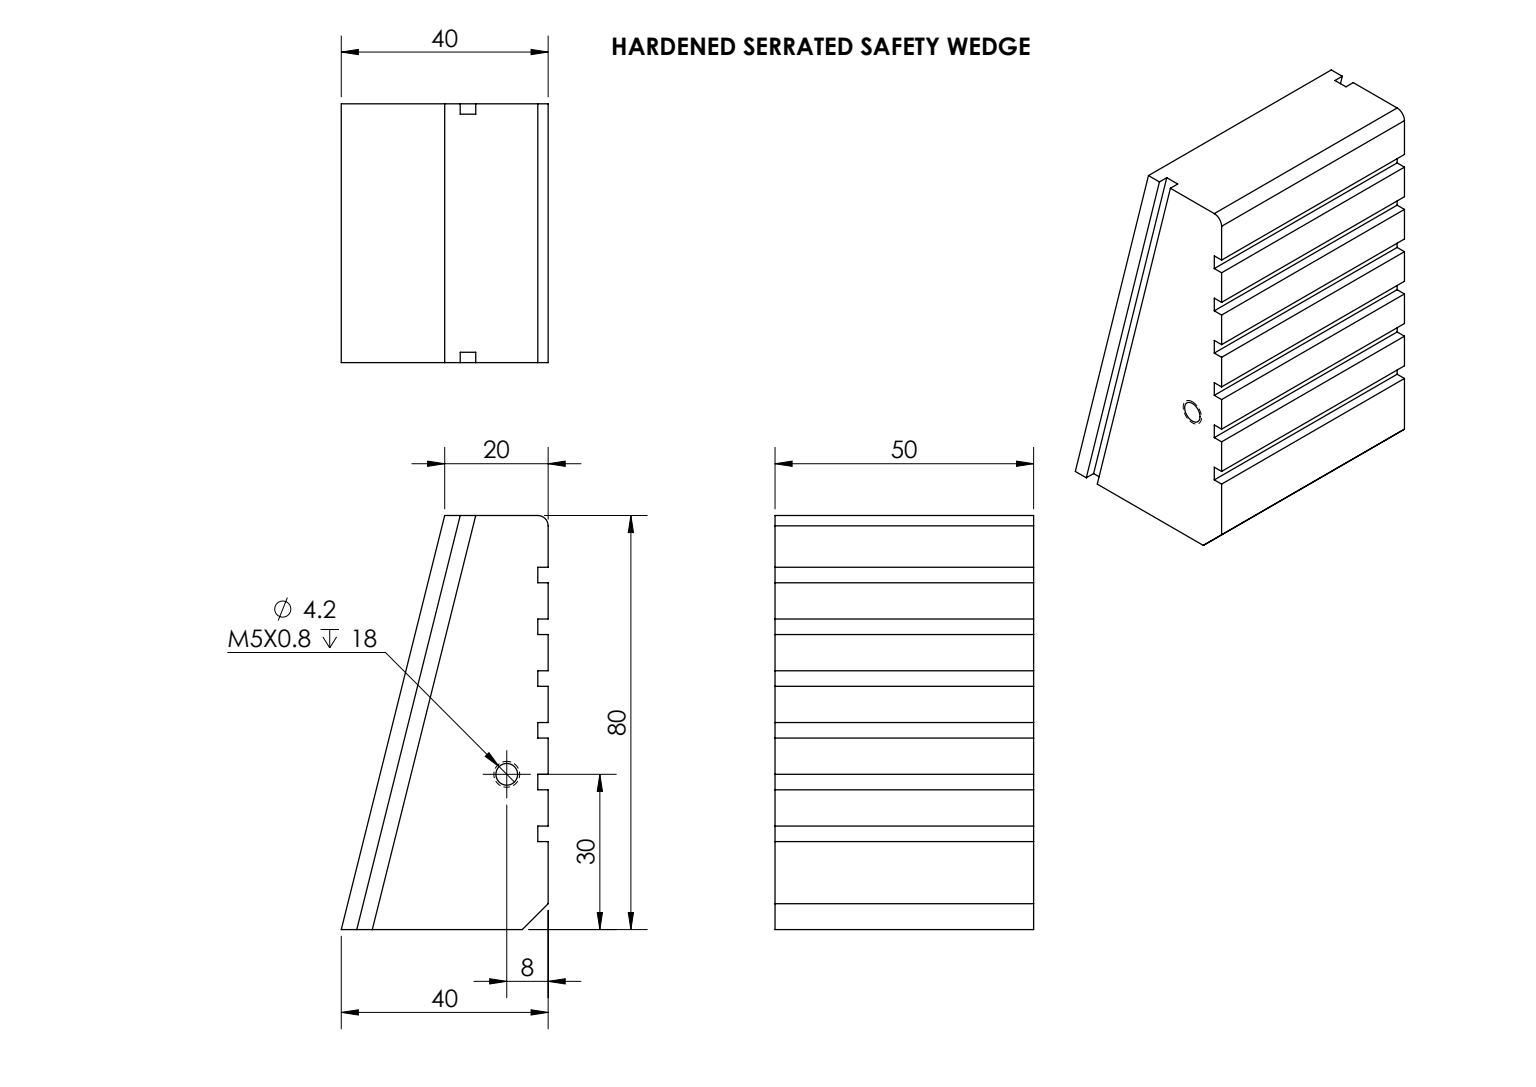
ISO-10303-21;
HEADER;
FILE_DESCRIPTION (('STEP AP214'),
    '1' );
FILE_NAME ('Hardened Serrated Safety Wedge.step',
    '2026-09-24T10:26:00',
    ( '' ),
    ( '' ),
    'SwSTEP 2.0',
    'SolidWorks 2026',
    '' );
FILE_SCHEMA (( 'AUTOMOTIVE_DESIGN' ));
ENDSEC;

DATA;
#10=ORIENTED_EDGE ( 'NONE', *, *, #2223, .T. ) ;
#11=CARTESIAN_POINT ( 'NONE',  ( 36.99999999999999289, 80.00000000000000000, -25.00000000000000000 ) ) ;
#20=DIRECTION ( 'NONE',  ( -1.000000000000000000, 0.000000000000000000, 0.000000000000000000 ) ) ;
#28=FILL_AREA_STYLE ('',( #13572 ) ) ;
#66=LINE ( 'NONE', #136, #7181 ) ;
#72=EDGE_CURVE ( 'NONE', #4842, #5455, #11044, .T. ) ;
#91=DIRECTION ( 'NONE',  ( -0.000000000000000000, -0.000000000000000000, -1.000000000000000000 ) ) ;
#92=ORIENTED_EDGE ( 'NONE', *, *, #1429, .T. ) ;
#97=LINE ( 'NONE', #11278, #533 ) ;
#101=DIRECTION ( 'NONE',  ( 0.000000000000000000, 0.000000000000000000, -1.000000000000000000 ) ) ;
#102=LINE ( 'NONE', #4701, #4263 ) ;
#121=ORIENTED_EDGE ( 'NONE', *, *, #9321, .T. ) ;
#122=DIRECTION ( 'NONE',  ( -0.000000000000000000, -1.000000000000000000, -0.000000000000000000 ) ) ;
#123=ADVANCED_FACE ( 'NONE', ( #3728 ), #1486, .F. ) ;
#124=DIRECTION ( 'NONE',  ( -1.000000000000000000, -1.224646799147353454E-16, 0.000000000000000000 ) ) ;
#126=ORIENTED_EDGE ( 'NONE', *, *, #8617, .F. ) ;
#136=CARTESIAN_POINT ( 'NONE',  ( 19.99999999999999645, 67.00000000000000000, -25.00000000000000000 ) ) ;
#157=AXIS2_PLACEMENT_3D ( 'NONE', #14374, #7610, #12245 ) ;
#161=EDGE_CURVE ( 'NONE', #1060, #1016, #5743, .T. ) ;
#164=ORIENTED_EDGE ( 'NONE', *, *, #6756, .F. ) ;
#166=VECTOR ( 'NONE', #2081, 1000.000000000000000 ) ;
#167=CARTESIAN_POINT ( 'NONE',  ( 0.000000000000000000, 0.000000000000000000, 0.000000000000000000 ) ) ;
#177=DIRECTION ( 'NONE',  ( 0.000000000000000000, 0.000000000000000000, -1.000000000000000000 ) ) ;
#181=VERTEX_POINT ( 'NONE', #10380 ) ;
#197=DIRECTION ( 'NONE',  ( -1.000000000000000000, -0.000000000000000000, -0.000000000000000000 ) ) ;
#209=ORIENTED_EDGE ( 'NONE', *, *, #6776, .T. ) ;
#210=CARTESIAN_POINT ( 'NONE',  ( 22.00000000000000355, 40.00000000000000711, 25.00000000000000000 ) ) ;
#211=ORIENTED_EDGE ( 'NONE', *, *, #12673, .T. ) ;
#223=VECTOR ( 'NONE', #6277, 1000.000000000000000 ) ;
#224=ORIENTED_EDGE ( 'NONE', *, *, #11005, .F. ) ;
#226=ORIENTED_EDGE ( 'NONE', *, *, #6230, .T. ) ;
#228=CARTESIAN_POINT ( 'NONE',  ( 22.00000000000000000, 67.00000000000000000, 25.00000000000000000 ) ) ;
#234=ORIENTED_EDGE ( 'NONE', *, *, #1565, .T. ) ;
#239=EDGE_CURVE ( 'NONE', #9259, #13438, #9577, .T. ) ;
#258=VECTOR ( 'NONE', #7960, 1000.000000000000000 ) ;
#273=FACE_OUTER_BOUND ( 'NONE', #4402, .T. ) ;
#286=ORIENTED_EDGE ( 'NONE', *, *, #14219, .T. ) ;
#294=FACE_OUTER_BOUND ( 'NONE', #7069, .T. ) ;
#297=CARTESIAN_POINT ( 'NONE',  ( 28.00000000000000355, 29.99999999999999645, -6.999999999999992006 ) ) ;
#298=PLANE ( 'NONE',  #9372 ) ;
#301=VECTOR ( 'NONE', #2565, 1000.000000000000000 ) ;
#305=EDGE_CURVE ( 'NONE', #1178, #14168, #3877, .T. ) ;
#311=EDGE_CURVE ( 'NONE', #7235, #651, #5038, .T. ) ;
#329=ORIENTED_EDGE ( 'NONE', *, *, #2055, .F. ) ;
#336=LINE ( 'NONE', #6016, #9990 ) ;
#337=VERTEX_POINT ( 'NONE', #12933 ) ;
#355=CARTESIAN_POINT ( 'NONE',  ( 20.00000000000000000, 70.00000000000000000, 25.00000000000000000 ) ) ;
#373=VERTEX_POINT ( 'NONE', #7643 ) ;
#402=CARTESIAN_POINT ( 'NONE',  ( 20.00000000000000000, 47.00000000000000000, -25.00000000000000000 ) ) ;
#407=DIRECTION ( 'NONE',  ( 0.000000000000000000, 0.000000000000000000, -1.000000000000000000 ) ) ;
#426=VECTOR ( 'NONE', #4169, 1000.000000000000114 ) ;
#429=EDGE_CURVE ( 'NONE', #1264, #5665, #1074, .T. ) ;
#434=VECTOR ( 'NONE', #1179, 1000.000000000000000 ) ;
#435=VERTEX_POINT ( 'NONE', #12201 ) ;
#448=LINE ( 'NONE', #1383, #301 ) ;
#485=CARTESIAN_POINT ( 'NONE',  ( 19.99999999999999645, 57.00000000000000000, 25.00000000000000000 ) ) ;
#509=LINE ( 'NONE', #9432, #9588 ) ;
#511=AXIS2_PLACEMENT_3D ( 'NONE', #2346, #91, #4566 ) ;
#513=LINE ( 'NONE', #8482, #11201 ) ;
#521=CARTESIAN_POINT ( 'NONE',  ( 28.00000000000000355, 29.99999999999999645, -5.738192700042120897 ) ) ;
#533=VECTOR ( 'NONE', #11200, 1000.000000000000000 ) ;
#538=ORIENTED_EDGE ( 'NONE', *, *, #8944, .T. ) ;
#553=FACE_OUTER_BOUND ( 'NONE', #9521, .T. ) ;
#560=LINE ( 'NONE', #11665, #13855 ) ;
#576=PLANE ( 'NONE',  #3995 ) ;
#587=DIRECTION ( 'NONE',  ( -0.2425356250363328581, 0.9701425001453318764, -0.000000000000000000 ) ) ;
#594=LINE ( 'NONE', #11851, #8147 ) ;
#612=ORIENTED_EDGE ( 'NONE', *, *, #11829, .T. ) ;
#618=FACE_OUTER_BOUND ( 'NONE', #7794, .T. ) ;
#634=ORIENTED_EDGE ( 'NONE', *, *, #1889, .T. ) ;
#649=ORIENTED_EDGE ( 'NONE', *, *, #239, .T. ) ;
#651=VERTEX_POINT ( 'NONE', #11316 ) ;
#654=DIRECTION ( 'NONE',  ( 0.7071067811865467956, -0.7071067811865483499, -0.000000000000000000 ) ) ;
#676=VECTOR ( 'NONE', #9454, 1000.000000000000000 ) ;
#678=VECTOR ( 'NONE', #13825, 1000.000000000000000 ) ;
#691=CARTESIAN_POINT ( 'NONE',  ( 30.10000000000000497, 29.99999999999999645, -6.999999999999992006 ) ) ;
#715=CARTESIAN_POINT ( 'NONE',  ( 20.00000000000000000, -5.510910596163090344E-15, 25.00000000000000000 ) ) ;
#718=DIRECTION ( 'NONE',  ( -1.000000000000000000, 0.000000000000000000, 0.000000000000000000 ) ) ;
#719=DIRECTION ( 'NONE',  ( -0.000000000000000000, 1.000000000000000000, 0.000000000000000000 ) ) ;
#721=VERTEX_POINT ( 'NONE', #10426 ) ;
#730=VECTOR ( 'NONE', #6841, 1000.000000000000000 ) ;
#736=ADVANCED_FACE ( 'NONE', ( #5952 ), #4871, .T. ) ;
#741=ORIENTED_EDGE ( 'NONE', *, *, #8946, .F. ) ;
#742=EDGE_CURVE ( 'NONE', #5183, #3543, #1654, .T. ) ;
#744=ORIENTED_EDGE ( 'NONE', *, *, #1270, .T. ) ;
#752=LINE ( 'NONE', #6297, #3942 ) ;
#755=DIRECTION ( 'NONE',  ( 0.9701425001453319874, 0.2425356250363328858, -0.000000000000000000 ) ) ;
#762=DIRECTION ( 'NONE',  ( 0.8571673007021134438, 1.049727191138620051E-16, -0.5150380749100522682 ) ) ;
#777=VERTEX_POINT ( 'NONE', #1804 ) ;
#785=ORIENTED_EDGE ( 'NONE', *, *, #8014, .F. ) ;
#789=FACE_OUTER_BOUND ( 'NONE', #1160, .T. ) ;
#806=PLANE ( 'NONE',  #7277 ) ;
#808=ORIENTED_EDGE ( 'NONE', *, *, #305, .F. ) ;
#809=DIRECTION ( 'NONE',  ( 0.000000000000000000, 0.000000000000000000, -1.000000000000000000 ) ) ;
#815=VERTEX_POINT ( 'NONE', #7418 ) ;
#844=CARTESIAN_POINT ( 'NONE',  ( 20.00000000000000000, 60.00000000000000711, -25.00000000000000000 ) ) ;
#864=CARTESIAN_POINT ( 'NONE',  ( 0.000000000000000000, 0.000000000000000000, 25.00000000000000000 ) ) ;
#869=CARTESIAN_POINT ( 'NONE',  ( 19.99999999999999645, 57.00000000000000000, -25.00000000000000000 ) ) ;
#871=VECTOR ( 'NONE', #14102, 1000.000000000000000 ) ;
#873=LINE ( 'NONE', #3165, #7989 ) ;
#874=CARTESIAN_POINT ( 'NONE',  ( 22.00000000000000355, 30.00000000000000711, 25.00000000000000000 ) ) ;
#882=CARTESIAN_POINT ( 'NONE',  ( 20.00000000000000355, 17.00000000000000000, 25.00000000000000000 ) ) ;
#890=VECTOR ( 'NONE', #3948, 1000.000000000000000 ) ;
#892=FACE_BOUND ( 'NONE', #3702, .T. ) ;
#895=ORIENTED_EDGE ( 'NONE', *, *, #5382, .T. ) ;
#905=EDGE_LOOP ( 'NONE', ( #9782, #10029, #10993, #1163 ) ) ;
#936=EDGE_CURVE ( 'NONE', #1368, #337, #11148, .T. ) ;
#939=ORIENTED_EDGE ( 'NONE', *, *, #7348, .T. ) ;
#941=VECTOR ( 'NONE', #3510, 1000.000000000000000 ) ;
#959=CARTESIAN_POINT ( 'NONE',  ( 56.99999999999997868, -8.673617379884035472E-16, -25.00000000000000000 ) ) ;
#975=PLANE ( 'NONE',  #9030 ) ;
#976=COLOUR_RGB ( '', 0.40784314, 0.44705882, 0.49803922) ;
#1001=ORIENTED_EDGE ( 'NONE', *, *, #8828, .F. ) ;
#1007=EDGE_CURVE ( 'NONE', #8772, #4305, #2374, .T. ) ;
#1014=VECTOR ( 'NONE', #5792, 1000.000000000000000 ) ;
#1016=VERTEX_POINT ( 'NONE', #13577 ) ;
#1024=ORIENTED_EDGE ( 'NONE', *, *, #3965, .T. ) ;
#1030=PLANE ( 'NONE',  #1314 ) ;
#1041=LINE ( 'NONE', #402, #1014 ) ;
#1042=ADVANCED_BREP_SHAPE_REPRESENTATION ( '', ( #6767, #11025 ), #6359 ) ;
#1060=VERTEX_POINT ( 'NONE', #6163 ) ;
#1061=DIRECTION ( 'NONE',  ( 0.000000000000000000, 0.000000000000000000, -1.000000000000000000 ) ) ;
#1073=VERTEX_POINT ( 'NONE', #6075 ) ;
#1074=LINE ( 'NONE', #9718, #12689 ) ;
#1108=LINE ( 'NONE', #3244, #10599 ) ;
#1120=ORIENTED_EDGE ( 'NONE', *, *, #4565, .T. ) ;
#1122=( NAMED_UNIT ( * ) SI_UNIT ( $, .STERADIAN. ) SOLID_ANGLE_UNIT ( ) );
#1127=AXIS2_PLACEMENT_3D ( 'NONE', #10215, #1359, #3582 ) ;
#1153=CARTESIAN_POINT ( 'NONE',  ( 20.00000000000000000, 60.00000000000000711, 25.00000000000000000 ) ) ;
#1160=EDGE_LOOP ( 'NONE', ( #13641, #4625, #1471, #1505 ) ) ;
#1163=ORIENTED_EDGE ( 'NONE', *, *, #13094, .F. ) ;
#1169=CARTESIAN_POINT ( 'NONE',  ( 22.00000000000000000, 70.00000000000000000, 25.00000000000000000 ) ) ;
#1178=VERTEX_POINT ( 'NONE', #7398 ) ;
#1179=DIRECTION ( 'NONE',  ( -1.000000000000000000, -0.000000000000000000, -0.000000000000000000 ) ) ;
#1187=CARTESIAN_POINT ( 'NONE',  ( 20.00000000000000000, -5.510910596163090344E-15, -25.00000000000000000 ) ) ;
#1214=AXIS2_PLACEMENT_3D ( 'NONE', #9472, #13943, #8363 ) ;
#1217=VERTEX_POINT ( 'NONE', #7543 ) ;
#1223=VECTOR ( 'NONE', #11410, 1000.000000000000000 ) ;
#1229=LINE ( 'NONE', #8834, #12194 ) ;
#1241=LINE ( 'NONE', #2558, #4227 ) ;
#1246=EDGE_LOOP ( 'NONE', ( #2231, #9201, #6977, #5095 ) ) ;
#1248=DIRECTION ( 'NONE',  ( -0.000000000000000000, 1.000000000000000000, -0.000000000000000000 ) ) ;
#1264=VERTEX_POINT ( 'NONE', #959 ) ;
#1270=EDGE_CURVE ( 'NONE', #10062, #435, #8650, .T. ) ;
#1290=SURFACE_STYLE_FILL_AREA ( #6856 ) ;
#1311=ORIENTED_EDGE ( 'NONE', *, *, #7811, .F. ) ;
#1313=EDGE_LOOP ( 'NONE', ( #3126, #4583, #612, #8364 ) ) ;
#1314=AXIS2_PLACEMENT_3D ( 'NONE', #9957, #12301, #13335 ) ;
#1322=CARTESIAN_POINT ( 'NONE',  ( 22.00000000000000000, 60.00000000000000711, 25.00000000000000000 ) ) ;
#1323=VECTOR ( 'NONE', #124, 1000.000000000000000 ) ;
#1359=DIRECTION ( 'NONE',  ( -0.000000000000000000, 1.000000000000000000, 0.000000000000000000 ) ) ;
#1361=PLANE ( 'NONE',  #11448 ) ;
#1368=VERTEX_POINT ( 'NONE', #11670 ) ;
#1382=MECHANICAL_DESIGN_GEOMETRIC_PRESENTATION_REPRESENTATION('',(#3971),#9336);
#1383=CARTESIAN_POINT ( 'NONE',  ( 22.00000000000000711, 20.00000000000000355, 25.00000000000000000 ) ) ;
#1388=EDGE_LOOP ( 'NONE', ( #2561, #11617, #939, #10546 ) ) ;
#1429=EDGE_CURVE ( 'NONE', #9259, #815, #12695, .T. ) ;
#1436=CARTESIAN_POINT ( 'NONE',  ( 20.00000000000000000, -5.510910596163090344E-15, -25.00000000000000000 ) ) ;
#1446=ADVANCED_FACE ( 'NONE', ( #10505 ), #13953, .T. ) ;
#1471=ORIENTED_EDGE ( 'NONE', *, *, #8427, .F. ) ;
#1486=CONICAL_SURFACE ( 'NONE', #7542, 2.100000000000000977, 1.029744258676656754 ) ;
#1505=ORIENTED_EDGE ( 'NONE', *, *, #12501, .F. ) ;
#1507=VERTEX_POINT ( 'NONE', #7353 ) ;
#1525=VERTEX_POINT ( 'NONE', #11830 ) ;
#1527=DIRECTION ( 'NONE',  ( -0.2425356250363328581, 0.9701425001453318764, 0.000000000000000000 ) ) ;
#1557=CARTESIAN_POINT ( 'NONE',  ( 20.00000000000000000, 60.00000000000000711, 25.00000000000000000 ) ) ;
#1563=VERTEX_POINT ( 'NONE', #6738 ) ;
#1565=EDGE_CURVE ( 'NONE', #5395, #6157, #7605, .T. ) ;
#1582=DIRECTION ( 'NONE',  ( -1.000000000000000000, 0.000000000000000000, 0.000000000000000000 ) ) ;
#1596=DIRECTION ( 'NONE',  ( -1.000000000000000000, 0.000000000000000000, -0.000000000000000000 ) ) ;
#1598=CARTESIAN_POINT ( 'NONE',  ( 20.00000000000000000, 47.00000000000000000, 25.00000000000000000 ) ) ;
#1600=CARTESIAN_POINT ( 'NONE',  ( 19.99999999999999645, 67.00000000000000000, 25.00000000000000000 ) ) ;
#1634=ORIENTED_EDGE ( 'NONE', *, *, #6804, .T. ) ;
#1639=CARTESIAN_POINT ( 'NONE',  ( 36.99999999999999289, 80.00000000000000000, -25.00000000000000000 ) ) ;
#1644=DIRECTION ( 'NONE',  ( 1.000000000000000000, 0.000000000000000000, 0.000000000000000000 ) ) ;
#1645=VERTEX_POINT ( 'NONE', #8115 ) ;
#1647=EDGE_CURVE ( 'NONE', #9523, #181, #102, .T. ) ;
#1654=LINE ( 'NONE', #12854, #2675 ) ;
#1661=LINE ( 'NONE', #6109, #10008 ) ;
#1673=CARTESIAN_POINT ( 'NONE',  ( 40.00000000000000711, 80.00000000000000000, 25.00000000000000000 ) ) ;
#1675=ORIENTED_EDGE ( 'NONE', *, *, #10881, .F. ) ;
#1680=CARTESIAN_POINT ( 'NONE',  ( 22.00000000000000000, 70.00000000000000000, 25.00000000000000000 ) ) ;
#1685=LINE ( 'NONE', #10684, #5641 ) ;
#1709=PRODUCT ( 'Hardened Serrated Safety Wedge', 'Hardened Serrated Safety Wedge', '', ( #3087 ) ) ;
#1716=CARTESIAN_POINT ( 'NONE',  ( 56.99999999999997868, -8.673617379884035472E-16, 23.00000000000000000 ) ) ;
#1722=VERTEX_POINT ( 'NONE', #12984 ) ;
#1723=CARTESIAN_POINT ( 'NONE',  ( 22.00000000000000000, 70.00000000000000000, 25.00000000000000000 ) ) ;
#1739=CARTESIAN_POINT ( 'NONE',  ( 33.99999999999998579, 80.00000000000000000, 23.00000000000000000 ) ) ;
#1742=CARTESIAN_POINT ( 'NONE',  ( 54.35294117647056567, -1.411764705882362358, 25.00000000000000000 ) ) ;
#1743=EDGE_CURVE ( 'NONE', #4861, #4373, #3896, .T. ) ;
#1745=EDGE_LOOP ( 'NONE', ( #6476, #4758, #12311, #5613 ) ) ;
#1748=DIRECTION ( 'NONE',  ( 0.000000000000000000, 0.000000000000000000, -1.000000000000000000 ) ) ;
#1755=CARTESIAN_POINT ( 'NONE',  ( 22.00000000000000711, 20.00000000000000355, -25.00000000000000000 ) ) ;
#1768=ORIENTED_EDGE ( 'NONE', *, *, #2005, .T. ) ;
#1793=CARTESIAN_POINT ( 'NONE',  ( 57.35294117647057277, -1.411764705882362358, -25.00000000000000000 ) ) ;
#1796=LINE ( 'NONE', #2827, #10774 ) ;
#1804=CARTESIAN_POINT ( 'NONE',  ( 22.00000000000000000, 67.00000000000000000, -25.00000000000000000 ) ) ;
#1809=ADVANCED_FACE ( 'NONE', ( #6293 ), #5056, .F. ) ;
#1815=LINE ( 'NONE', #6338, #5328 ) ;
#1826=LINE ( 'NONE', #1598, #6288 ) ;
#1834=VECTOR ( 'NONE', #2821, 1000.000000000000227 ) ;
#1836=ORIENTED_EDGE ( 'NONE', *, *, #2559, .F. ) ;
#1852=CARTESIAN_POINT ( 'NONE',  ( 57.35294117647057277, -1.411764705882362358, -25.00000000000000000 ) ) ;
#1855=LINE ( 'NONE', #7254, #8774 ) ;
#1878=ORIENTED_EDGE ( 'NONE', *, *, #12626, .F. ) ;
#1883=PLANE ( 'NONE',  #3706 ) ;
#1886=CARTESIAN_POINT ( 'NONE',  ( 57.35294117647057277, -1.411764705882362358, 23.00000000000000000 ) ) ;
#1887=CARTESIAN_POINT ( 'NONE',  ( 20.00000000000000000, 27.00000000000000355, 25.00000000000000000 ) ) ;
#1889=EDGE_CURVE ( 'NONE', #1368, #8027, #8777, .T. ) ;
#1907=ORIENTED_EDGE ( 'NONE', *, *, #5733, .T. ) ;
#1909=ADVANCED_FACE ( 'NONE', ( #5485 ), #13413, .F. ) ;
#1953=AXIS2_PLACEMENT_3D ( 'NONE', #7106, #11430, #5005 ) ;
#1974=CARTESIAN_POINT ( 'NONE',  ( 20.00000000000000000, -5.510910596163090344E-15, -25.00000000000000000 ) ) ;
#1975=CARTESIAN_POINT ( 'NONE',  ( 20.00000000000000000, 78.00000000000000000, -25.00000000000000000 ) ) ;
#1977=FACE_OUTER_BOUND ( 'NONE', #8291, .T. ) ;
#1983=EDGE_CURVE ( 'NONE', #12581, #2621, #1241, .T. ) ;
#2005=EDGE_CURVE ( 'NONE', #9291, #5102, #9129, .T. ) ;
#2008=ORIENTED_EDGE ( 'NONE', *, *, #2079, .T. ) ;
#2009=ORIENTED_EDGE ( 'NONE', *, *, #936, .T. ) ;
#2016=EDGE_CURVE ( 'NONE', #1217, #11907, #9581, .T. ) ;
#2027=VECTOR ( 'NONE', #13139, 1000.000000000000000 ) ;
#2037=PLANE ( 'NONE',  #6947 ) ;
#2055=EDGE_CURVE ( 'NONE', #5455, #14165, #5973, .T. ) ;
#2064=EDGE_CURVE ( 'NONE', #3193, #1507, #9654, .T. ) ;
#2069=LINE ( 'NONE', #1187, #2027 ) ;
#2071=VECTOR ( 'NONE', #122, 1000.000000000000000 ) ;
#2079=EDGE_CURVE ( 'NONE', #3573, #12564, #513, .T. ) ;
#2081=DIRECTION ( 'NONE',  ( -0.000000000000000000, -0.000000000000000000, 1.000000000000000000 ) ) ;
#2084=EDGE_CURVE ( 'NONE', #10580, #1563, #11781, .T. ) ;
#2085=EDGE_CURVE ( 'NONE', #6341, #10817, #1826, .T. ) ;
#2090=EDGE_CURVE ( 'NONE', #9523, #5064, #594, .T. ) ;
#2093=DIRECTION ( 'NONE',  ( 0.000000000000000000, 0.000000000000000000, -1.000000000000000000 ) ) ;
#2098=DIRECTION ( 'NONE',  ( 0.000000000000000000, 0.000000000000000000, -1.000000000000000000 ) ) ;
#2100=VECTOR ( 'NONE', #2190, 1000.000000000000000 ) ;
#2142=CARTESIAN_POINT ( 'NONE',  ( 22.00000000000000000, 70.00000000000000000, -25.00000000000000000 ) ) ;
#2152=DIRECTION ( 'NONE',  ( 0.000000000000000000, 0.000000000000000000, -1.000000000000000000 ) ) ;
#2184=CIRCLE ( 'NONE', #4525, 2.100000000000000977 ) ;
#2190=DIRECTION ( 'NONE',  ( -0.000000000000000000, -1.000000000000000000, -0.000000000000000000 ) ) ;
#2214=VECTOR ( 'NONE', #1061, 1000.000000000000000 ) ;
#2220=CARTESIAN_POINT ( 'NONE',  ( 12.50000000000002132, 12.49999999999999289, -25.00000000000000000 ) ) ;
#2223=EDGE_CURVE ( 'NONE', #4126, #4373, #13031, .T. ) ;
#2231=ORIENTED_EDGE ( 'NONE', *, *, #2064, .F. ) ;
#2232=FACE_OUTER_BOUND ( 'NONE', #11849, .T. ) ;
#2256=CARTESIAN_POINT ( 'NONE',  ( 22.00000000000000000, 70.00000000000000000, 25.00000000000000000 ) ) ;
#2258=EDGE_CURVE ( 'NONE', #5183, #9564, #3081, .T. ) ;
#2275=CARTESIAN_POINT ( 'NONE',  ( 20.00000000000000000, 5.000000000000000000, 25.00000000000000000 ) ) ;
#2287=CARTESIAN_POINT ( 'NONE',  ( 20.00000000000000000, 27.00000000000000355, 25.00000000000000000 ) ) ;
#2314=LINE ( 'NONE', #4532, #1323 ) ;
#2324=LINE ( 'NONE', #6775, #12846 ) ;
#2327=VECTOR ( 'NONE', #2940, 1000.000000000000000 ) ;
#2346=CARTESIAN_POINT ( 'NONE',  ( 28.00000000000000355, 29.99999999999999645, -25.00000000000000000 ) ) ;
#2364=ORIENTED_EDGE ( 'NONE', *, *, #11159, .T. ) ;
#2374=LINE ( 'NONE', #3482, #2214 ) ;
#2377=CARTESIAN_POINT ( 'NONE',  ( 22.00000000000000355, 30.00000000000000711, 25.00000000000000000 ) ) ;
#2378=CARTESIAN_POINT ( 'NONE',  ( 20.00000000000000000, 37.00000000000000711, 25.00000000000000000 ) ) ;
#2379=LINE ( 'NONE', #4720, #7432 ) ;
#2389=ORIENTED_EDGE ( 'NONE', *, *, #9189, .F. ) ;
#2433=DIRECTION ( 'NONE',  ( -0.000000000000000000, 0.000000000000000000, 1.000000000000000000 ) ) ;
#2435=ORIENTED_EDGE ( 'NONE', *, *, #14124, .T. ) ;
#2453=EDGE_LOOP ( 'NONE', ( #7931, #9555, #808, #10717 ) ) ;
#2470=LINE ( 'NONE', #2546, #4243 ) ;
#2476=ORIENTED_EDGE ( 'NONE', *, *, #13211, .F. ) ;
#2480=CARTESIAN_POINT ( 'NONE',  ( 22.00000000000000000, 70.00000000000000000, -25.00000000000000000 ) ) ;
#2489=CARTESIAN_POINT ( 'NONE',  ( 20.00000000000000355, 50.00000000000000000, 25.00000000000000000 ) ) ;
#2492=EDGE_LOOP ( 'NONE', ( #3472, #7425, #6478, #3054 ) ) ;
#2498=ORIENTED_EDGE ( 'NONE', *, *, #7318, .T. ) ;
#2527=DIRECTION ( 'NONE',  ( -0.2425356250363328581, 0.9701425001453318764, 0.000000000000000000 ) ) ;
#2546=CARTESIAN_POINT ( 'NONE',  ( 20.00000000000000355, 30.00000000000000711, 25.00000000000000000 ) ) ;
#2558=CARTESIAN_POINT ( 'NONE',  ( 20.00000000000000000, 60.00000000000000711, -25.00000000000000000 ) ) ;
#2559=EDGE_CURVE ( 'NONE', #6341, #10062, #12622, .T. ) ;
#2561=ORIENTED_EDGE ( 'NONE', *, *, #10392, .F. ) ;
#2565=DIRECTION ( 'NONE',  ( -0.000000000000000000, 1.000000000000000000, -0.000000000000000000 ) ) ;
#2570=ORIENTED_EDGE ( 'NONE', *, *, #2223, .F. ) ;
#2577=ORIENTED_EDGE ( 'NONE', *, *, #8273, .T. ) ;
#2578=DIRECTION ( 'NONE',  ( -1.000000000000000000, 0.000000000000000000, -0.000000000000000000 ) ) ;
#2585=PLANE ( 'NONE',  #1953 ) ;
#2597=CARTESIAN_POINT ( 'NONE',  ( 20.00000000000000355, 40.00000000000000711, -25.00000000000000000 ) ) ;
#2600=VECTOR ( 'NONE', #13843, 1000.000000000000000 ) ;
#2613=DIRECTION ( 'NONE',  ( 0.000000000000000000, -1.000000000000000000, 0.000000000000000000 ) ) ;
#2621=VERTEX_POINT ( 'NONE', #844 ) ;
#2638=DIRECTION ( 'NONE',  ( 1.000000000000000000, 0.000000000000000000, 0.000000000000000000 ) ) ;
#2646=EDGE_CURVE ( 'NONE', #435, #5824, #8675, .T. ) ;
#2663=VECTOR ( 'NONE', #10225, 1000.000000000000000 ) ;
#2675=VECTOR ( 'NONE', #3787, 1000.000000000000000 ) ;
#2680=EDGE_CURVE ( 'NONE', #1178, #5665, #8815, .T. ) ;
#2694=LINE ( 'NONE', #715, #5098 ) ;
#2707=DIRECTION ( 'NONE',  ( -0.000000000000000000, 0.000000000000000000, 1.000000000000000000 ) ) ;
#2731=ORIENTED_EDGE ( 'NONE', *, *, #9196, .T. ) ;
#2735=ORIENTED_EDGE ( 'NONE', *, *, #9535, .T. ) ;
#2754=EDGE_LOOP ( 'NONE', ( #12609, #12486, #4903, #9949, #10444, #785, #12523, #13410, #5775, #4321, #6309, #3499, #649, #13958, #10226, #1836, #226, #164, #12811, #12934, #121, #8467, #8808, #8615, #11419, #2831, #2476, #7743, #10745, #7634 ) ) ;
#2757=AXIS2_PLACEMENT_3D ( 'NONE', #4083, #13073, #6319 ) ;
#2760=VECTOR ( 'NONE', #6987, 1000.000000000000000 ) ;
#2765=PLANE ( 'NONE',  #4916 ) ;
#2770=EDGE_CURVE ( 'NONE', #10977, #12581, #2379, .T. ) ;
#2776=VECTOR ( 'NONE', #10811, 1000.000000000000000 ) ;
#2787=CARTESIAN_POINT ( 'NONE',  ( 22.00000000000000355, 30.00000000000000711, -25.00000000000000000 ) ) ;
#2805=EDGE_CURVE ( 'NONE', #12241, #7901, #10264, .T. ) ;
#2821=DIRECTION ( 'NONE',  ( -0.2425356250363328581, 0.9701425001453318764, -0.000000000000000000 ) ) ;
#2827=CARTESIAN_POINT ( 'NONE',  ( 60.00000000000000000, -6.123233995736768255E-16, -23.00000000000000000 ) ) ;
#2831=ORIENTED_EDGE ( 'NONE', *, *, #4707, .F. ) ;
#2846=CARTESIAN_POINT ( 'NONE',  ( 60.00000000000000000, -6.123233995736768255E-16, -25.00000000000000000 ) ) ;
#2859=CARTESIAN_POINT ( 'NONE',  ( 25.90000000000000213, 29.99999999999999645, -25.00000000000000000 ) ) ;
#2867=DIRECTION ( 'NONE',  ( 0.000000000000000000, 0.000000000000000000, -1.000000000000000000 ) ) ;
#2873=MECHANICAL_DESIGN_GEOMETRIC_PRESENTATION_REPRESENTATION('',(#5426),#12446);
#2904=VECTOR ( 'NONE', #4860, 1000.000000000000000 ) ;
#2907=CARTESIAN_POINT ( 'NONE',  ( 20.00000000000000000, -5.510910596163090344E-15, -25.00000000000000000 ) ) ;
#2922=DIRECTION ( 'NONE',  ( -1.000000000000000000, -0.000000000000000000, -0.000000000000000000 ) ) ;
#2930=FACE_OUTER_BOUND ( 'NONE', #10865, .T. ) ;
#2933=PLANE ( 'NONE',  #9775 ) ;
#2940=DIRECTION ( 'NONE',  ( -0.000000000000000000, -1.000000000000000000, -0.000000000000000000 ) ) ;
#2961=LINE ( 'NONE', #10633, #4986 ) ;
#2978=LINE ( 'NONE', #7347, #9045 ) ;
#2981=DIRECTION ( 'NONE',  ( 1.000000000000000000, 1.224646799147353454E-16, -0.000000000000000000 ) ) ;
#2983=CARTESIAN_POINT ( 'NONE',  ( 20.00000000000000355, 30.00000000000000711, 25.00000000000000000 ) ) ;
#2994=CARTESIAN_POINT ( 'NONE',  ( 20.00000000000000355, 17.00000000000000000, -25.00000000000000000 ) ) ;
#2997=ADVANCED_FACE ( 'NONE', ( #6579 ), #9808, .T. ) ;
#2998=EDGE_CURVE ( 'NONE', #1264, #7901, #10715, .T. ) ;
#3029=FACE_OUTER_BOUND ( 'NONE', #9225, .T. ) ;
#3039=ADVANCED_FACE ( 'NONE', ( #10097 ), #6654, .T. ) ;
#3040=ADVANCED_FACE ( 'NONE', ( #4417 ), #1030, .F. ) ;
#3043=LINE ( 'NONE', #4073, #9736 ) ;
#3054=ORIENTED_EDGE ( 'NONE', *, *, #13277, .F. ) ;
#3062=LINE ( 'NONE', #1739, #6317 ) ;
#3081=LINE ( 'NONE', #13240, #10258 ) ;
#3087=PRODUCT_CONTEXT ( 'NONE', #9795, 'mechanical' ) ;
#3100=LINE ( 'NONE', #13255, #13131 ) ;
#3126=ORIENTED_EDGE ( 'NONE', *, *, #2085, .F. ) ;
#3127=FACE_OUTER_BOUND ( 'NONE', #11935, .T. ) ;
#3131=EDGE_LOOP ( 'NONE', ( #7315, #5168, #9079, #14380, #126, #4095, #11671, #3360, #2498, #9694, #10895, #5389 ) ) ;
#3135=ORIENTED_EDGE ( 'NONE', *, *, #6230, .F. ) ;
#3140=DIRECTION ( 'NONE',  ( 0.000000000000000000, -1.000000000000000000, 0.000000000000000000 ) ) ;
#3162=EDGE_CURVE ( 'NONE', #373, #1264, #3043, .T. ) ;
#3165=CARTESIAN_POINT ( 'NONE',  ( 20.00000000000000000, -5.510910596163090344E-15, -25.00000000000000000 ) ) ;
#3169=DIRECTION ( 'NONE',  ( -1.000000000000000000, 0.000000000000000000, -0.000000000000000000 ) ) ;
#3170=VERTEX_POINT ( 'NONE', #8352 ) ;
#3173=CARTESIAN_POINT ( 'NONE',  ( 22.00000000000000355, 37.00000000000000711, 25.00000000000000000 ) ) ;
#3193=VERTEX_POINT ( 'NONE', #691 ) ;
#3201=DIRECTION ( 'NONE',  ( 0.000000000000000000, -0.000000000000000000, -1.000000000000000000 ) ) ;
#3224=LINE ( 'NONE', #869, #9413 ) ;
#3235=CARTESIAN_POINT ( 'NONE',  ( 22.00000000000000355, 50.00000000000000000, 25.00000000000000000 ) ) ;
#3244=CARTESIAN_POINT ( 'NONE',  ( 22.00000000000000000, 57.00000000000000000, 25.00000000000000000 ) ) ;
#3263=ORIENTED_EDGE ( 'NONE', *, *, #12673, .F. ) ;
#3265=EDGE_LOOP ( 'NONE', ( #10728, #1907, #5085, #7095 ) ) ;
#3278=AXIS2_PLACEMENT_3D ( 'NONE', #8415, #9670, #13047 ) ;
#3280=ADVANCED_FACE ( 'NONE', ( #13207 ), #11072, .T. ) ;
#3288=LINE ( 'NONE', #12492, #11902 ) ;
#3298=EDGE_CURVE ( 'NONE', #4830, #14165, #2069, .T. ) ;
#3308=DIRECTION ( 'NONE',  ( 0.9701425001453319874, 0.2425356250363328858, 0.000000000000000000 ) ) ;
#3323=LINE ( 'NONE', #2220, #5450 ) ;
#3324=ORIENTED_EDGE ( 'NONE', *, *, #4531, .F. ) ;
#3337=DIRECTION ( 'NONE',  ( -0.2425356250363328581, 0.9701425001453318764, 0.000000000000000000 ) ) ;
#3347=CARTESIAN_POINT ( 'NONE',  ( 19.99999999999999645, 57.00000000000000000, 25.00000000000000000 ) ) ;
#3360=ORIENTED_EDGE ( 'NONE', *, *, #4681, .F. ) ;
#3364=ORIENTED_EDGE ( 'NONE', *, *, #9327, .T. ) ;
#3394=ORIENTED_EDGE ( 'NONE', *, *, #10742, .T. ) ;
#3396=CARTESIAN_POINT ( 'NONE',  ( 20.00000000000000000, 80.00000000000000000, 25.00000000000000000 ) ) ;
#3443=ORIENTED_EDGE ( 'NONE', *, *, #13537, .F. ) ;
#3445=ORIENTED_EDGE ( 'NONE', *, *, #5382, .F. ) ;
#3457=PLANE ( 'NONE',  #3704 ) ;
#3472=ORIENTED_EDGE ( 'NONE', *, *, #5559, .F. ) ;
#3477=PLANE ( 'NONE',  #11503 ) ;
#3481=VECTOR ( 'NONE', #11583, 1000.000000000000000 ) ;
#3482=CARTESIAN_POINT ( 'NONE',  ( 20.00000000000000355, 40.00000000000000711, 25.00000000000000000 ) ) ;
#3494=AXIS2_PLACEMENT_3D ( 'NONE', #1742, #9568, #4014 ) ;
#3499=ORIENTED_EDGE ( 'NONE', *, *, #10742, .F. ) ;
#3506=FACE_OUTER_BOUND ( 'NONE', #5037, .T. ) ;
#3510=DIRECTION ( 'NONE',  ( 0.000000000000000000, 0.000000000000000000, -1.000000000000000000 ) ) ;
#3538=AXIS2_PLACEMENT_3D ( 'NONE', #3812, #14322, #11695 ) ;
#3543=VERTEX_POINT ( 'NONE', #14179 ) ;
#3552=DIRECTION ( 'NONE',  ( 1.000000000000000000, 0.000000000000000000, -0.000000000000000000 ) ) ;
#3573=VERTEX_POINT ( 'NONE', #14319 ) ;
#3582=DIRECTION ( 'NONE',  ( 0.000000000000000000, -0.000000000000000000, 1.000000000000000000 ) ) ;
#3588=AXIS2_PLACEMENT_3D ( 'NONE', #8981, #5408, #12220 ) ;
#3619=EDGE_CURVE ( 'NONE', #4830, #337, #12114, .T. ) ;
#3646=LINE ( 'NONE', #4737, #12617 ) ;
#3648=LINE ( 'NONE', #1436, #6034 ) ;
#3661=ORIENTED_EDGE ( 'NONE', *, *, #4029, .T. ) ;
#3698=CARTESIAN_POINT ( 'NONE',  ( 22.00000000000000355, 47.00000000000000000, 25.00000000000000000 ) ) ;
#3702=EDGE_LOOP ( 'NONE', ( #4228, #12719 ) ) ;
#3704=AXIS2_PLACEMENT_3D ( 'NONE', #13832, #7831, #3804 ) ;
#3706=AXIS2_PLACEMENT_3D ( 'NONE', #9926, #3140, #3201 ) ;
#3718=CARTESIAN_POINT ( 'NONE',  ( 20.00000000000000355, 40.00000000000000711, 25.00000000000000000 ) ) ;
#3725=LINE ( 'NONE', #7138, #8206 ) ;
#3728=FACE_OUTER_BOUND ( 'NONE', #8959, .T. ) ;
#3746=ORIENTED_EDGE ( 'NONE', *, *, #429, .T. ) ;
#3767=AXIS2_PLACEMENT_3D ( 'NONE', #3929, #7278, #11755 ) ;
#3773=CARTESIAN_POINT ( 'NONE',  ( 25.90000000000000213, 29.99999999999999645, -6.999999999999992006 ) ) ;
#3783=ORIENTED_EDGE ( 'NONE', *, *, #2005, .F. ) ;
#3787=DIRECTION ( 'NONE',  ( 0.000000000000000000, 0.000000000000000000, -1.000000000000000000 ) ) ;
#3789=ADVANCED_FACE ( 'NONE', ( #10486 ), #2585, .F. ) ;
#3804=DIRECTION ( 'NONE',  ( 0.000000000000000000, -0.000000000000000000, -1.000000000000000000 ) ) ;
#3806=ORIENTED_EDGE ( 'NONE', *, *, #3298, .F. ) ;
#3812=CARTESIAN_POINT ( 'NONE',  ( 60.00000000000000000, -6.123233995736768255E-16, 25.00000000000000000 ) ) ;
#3814=FACE_OUTER_BOUND ( 'NONE', #9176, .T. ) ;
#3837=LINE ( 'NONE', #4997, #676 ) ;
#3877=LINE ( 'NONE', #1673, #5911 ) ;
#3883=DIRECTION ( 'NONE',  ( 0.000000000000000000, 0.000000000000000000, -1.000000000000000000 ) ) ;
#3896=LINE ( 'NONE', #12739, #12186 ) ;
#3913=EDGE_LOOP ( 'NONE', ( #14433, #10649, #12146, #1878 ) ) ;
#3919=VECTOR ( 'NONE', #5955, 1000.000000000000000 ) ;
#3923=EDGE_CURVE ( 'NONE', #12157, #3193, #1855, .T. ) ;
#3924=LINE ( 'NONE', #2597, #2904 ) ;
#3929=CARTESIAN_POINT ( 'NONE',  ( 19.99999999999999645, 67.00000000000000000, 25.00000000000000000 ) ) ;
#3942=VECTOR ( 'NONE', #9599, 1000.000000000000000 ) ;
#3946=CIRCLE ( 'NONE', #10711, 2.100000000000000977 ) ;
#3948=DIRECTION ( 'NONE',  ( 1.000000000000000000, 0.000000000000000000, 0.000000000000000000 ) ) ;
#3965=EDGE_CURVE ( 'NONE', #3170, #9934, #5143, .T. ) ;
#3967=ORIENTED_EDGE ( 'NONE', *, *, #72, .F. ) ;
#3971=STYLED_ITEM ( 'NONE', ( #12209 ), #6767 ) ;
#3995=AXIS2_PLACEMENT_3D ( 'NONE', #5176, #10738, #5250 ) ;
#4007=CARTESIAN_POINT ( 'NONE',  ( 20.00000000000000000, 70.00000000000000000, 25.00000000000000000 ) ) ;
#4014=DIRECTION ( 'NONE',  ( 0.2425356250363328581, -0.9701425001453318764, 0.000000000000000000 ) ) ;
#4029=EDGE_CURVE ( 'NONE', #5022, #8001, #5066, .T. ) ;
#4037=CARTESIAN_POINT ( 'NONE',  ( 22.00000000000000000, 57.00000000000000000, -25.00000000000000000 ) ) ;
#4039=SHAPE_DEFINITION_REPRESENTATION ( #8348, #5343 ) ;
#4043=ORIENTED_EDGE ( 'NONE', *, *, #311, .F. ) ;
#4070=EDGE_CURVE ( 'NONE', #8001, #1525, #11284, .T. ) ;
#4073=CARTESIAN_POINT ( 'NONE',  ( 56.99999999999997868, -9.797174393178845379E-16, 25.00000000000000000 ) ) ;
#4083=CARTESIAN_POINT ( 'NONE',  ( 22.00000000000000355, 30.00000000000000711, 25.00000000000000000 ) ) ;
#4095=ORIENTED_EDGE ( 'NONE', *, *, #5830, .F. ) ;
#4103=CARTESIAN_POINT ( 'NONE',  ( 19.99999999999999645, 67.00000000000000000, 25.00000000000000000 ) ) ;
#4126=VERTEX_POINT ( 'NONE', #7609 ) ;
#4150=CARTESIAN_POINT ( 'NONE',  ( 22.00000000000000711, 17.00000000000000000, 25.00000000000000000 ) ) ;
#4163=CARTESIAN_POINT ( 'NONE',  ( 60.00000000000000000, -6.123233995736768255E-16, 25.00000000000000000 ) ) ;
#4169=DIRECTION ( 'NONE',  ( -0.2425356250363328581, 0.9701425001453318764, 0.000000000000000000 ) ) ;
#4212=DIRECTION ( 'NONE',  ( -0.000000000000000000, 1.000000000000000000, 0.000000000000000000 ) ) ;
#4219=CARTESIAN_POINT ( 'NONE',  ( 54.35294117647056567, -1.411764705882362358, -25.00000000000000000 ) ) ;
#4227=VECTOR ( 'NONE', #11402, 1000.000000000000000 ) ;
#4228=ORIENTED_EDGE ( 'NONE', *, *, #11919, .F. ) ;
#4236=EDGE_CURVE ( 'NONE', #1217, #777, #12455, .T. ) ;
#4243=VECTOR ( 'NONE', #11459, 1000.000000000000000 ) ;
#4244=AXIS2_PLACEMENT_3D ( 'NONE', #7611, #2152, #20 ) ;
#4263=VECTOR ( 'NONE', #4633, 1000.000000000000000 ) ;
#4277=DIRECTION ( 'NONE',  ( -1.000000000000000000, 0.000000000000000000, -0.000000000000000000 ) ) ;
#4284=LINE ( 'NONE', #2142, #8474 ) ;
#4305=VERTEX_POINT ( 'NONE', #10837 ) ;
#4309=APPLICATION_CONTEXT ( 'automotive_design' ) ;
#4321=ORIENTED_EDGE ( 'NONE', *, *, #6443, .F. ) ;
#4351=LINE ( 'NONE', #2489, #1223 ) ;
#4360=VECTOR ( 'NONE', #8651, 1000.000000000000000 ) ;
#4373=VERTEX_POINT ( 'NONE', #7323 ) ;
#4402=EDGE_LOOP ( 'NONE', ( #224, #2364, #6078, #8375 ) ) ;
#4404=ADVANCED_FACE ( 'NONE', ( #3029 ), #13123, .F. ) ;
#4408=ORIENTED_EDGE ( 'NONE', *, *, #2646, .T. ) ;
#4413=DIRECTION ( 'NONE',  ( -0.000000000000000000, -1.000000000000000000, -0.000000000000000000 ) ) ;
#4417=FACE_OUTER_BOUND ( 'NONE', #1745, .T. ) ;
#4448=EDGE_LOOP ( 'NONE', ( #9190, #11549, #7257, #10824 ) ) ;
#4493=ORIENTED_EDGE ( 'NONE', *, *, #8944, .F. ) ;
#4521=DIRECTION ( 'NONE',  ( 0.000000000000000000, -0.000000000000000000, 1.000000000000000000 ) ) ;
#4525=AXIS2_PLACEMENT_3D ( 'NONE', #8204, #7028, #13716 ) ;
#4531=EDGE_CURVE ( 'NONE', #10817, #4305, #873, .T. ) ;
#4532=CARTESIAN_POINT ( 'NONE',  ( 60.00000000000000000, -6.123233995736768255E-16, 23.00000000000000000 ) ) ;
#4543=DIRECTION ( 'NONE',  ( 1.000000000000000000, 0.000000000000000000, 0.000000000000000000 ) ) ;
#4547=EDGE_CURVE ( 'NONE', #6762, #5687, #4557, .T. ) ;
#4557=LINE ( 'NONE', #10019, #10820 ) ;
#4565=EDGE_CURVE ( 'NONE', #7705, #5395, #8918, .T. ) ;
#4566=DIRECTION ( 'NONE',  ( -1.000000000000000000, 0.000000000000000000, 0.000000000000000000 ) ) ;
#4583=ORIENTED_EDGE ( 'NONE', *, *, #2559, .T. ) ;
#4625=ORIENTED_EDGE ( 'NONE', *, *, #8617, .T. ) ;
#4633=DIRECTION ( 'NONE',  ( 0.000000000000000000, 0.000000000000000000, -1.000000000000000000 ) ) ;
#4634=AXIS2_PLACEMENT_3D ( 'NONE', #1322, #2578, #2433 ) ;
#4669=FILL_AREA_STYLE_COLOUR ( '', #10254 ) ;
#4671=DIRECTION ( 'NONE',  ( 0.000000000000000000, 0.000000000000000000, -1.000000000000000000 ) ) ;
#4672=VECTOR ( 'NONE', #10448, 1000.000000000000000 ) ;
#4680=VERTEX_POINT ( 'NONE', #2480 ) ;
#4681=EDGE_CURVE ( 'NONE', #14168, #3573, #7075, .T. ) ;
#4686=CARTESIAN_POINT ( 'NONE',  ( 20.00000000000000000, 80.00000000000000000, 25.00000000000000000 ) ) ;
#4689=FACE_OUTER_BOUND ( 'NONE', #4905, .T. ) ;
#4701=CARTESIAN_POINT ( 'NONE',  ( 19.99999999999999645, 67.00000000000000000, 25.00000000000000000 ) ) ;
#4707=EDGE_CURVE ( 'NONE', #4842, #9976, #6795, .T. ) ;
#4718=LINE ( 'NONE', #11740, #1834 ) ;
#4720=CARTESIAN_POINT ( 'NONE',  ( 22.00000000000000000, 60.00000000000000711, -25.00000000000000000 ) ) ;
#4737=CARTESIAN_POINT ( 'NONE',  ( 33.99999999999998579, 80.00000000000000000, -25.00000000000000000 ) ) ;
#4753=DIRECTION ( 'NONE',  ( -0.000000000000000000, 1.000000000000000000, -0.000000000000000000 ) ) ;
#4755=CARTESIAN_POINT ( 'NONE',  ( 56.99999999999997868, -9.797174393178845379E-16, 25.00000000000000000 ) ) ;
#4758=ORIENTED_EDGE ( 'NONE', *, *, #7735, .T. ) ;
#4762=VECTOR ( 'NONE', #7302, 1000.000000000000000 ) ;
#4767=ORIENTED_EDGE ( 'NONE', *, *, #4707, .T. ) ;
#4785=ADVANCED_FACE ( 'NONE', ( #9508 ), #10872, .F. ) ;
#4818=LINE ( 'NONE', #7074, #12605 ) ;
#4825=CARTESIAN_POINT ( 'NONE',  ( 22.00000000000000355, 47.00000000000000000, 25.00000000000000000 ) ) ;
#4830=VERTEX_POINT ( 'NONE', #11008 ) ;
#4842=VERTEX_POINT ( 'NONE', #5451 ) ;
#4845=ORIENTED_EDGE ( 'NONE', *, *, #14443, .T. ) ;
#4860=DIRECTION ( 'NONE',  ( -1.000000000000000000, -0.000000000000000000, -0.000000000000000000 ) ) ;
#4861=VERTEX_POINT ( 'NONE', #2787 ) ;
#4871=PLANE ( 'NONE',  #5244 ) ;
#4882=CARTESIAN_POINT ( 'NONE',  ( 22.00000000000000355, 30.00000000000000711, 25.00000000000000000 ) ) ;
#4888=ORIENTED_EDGE ( 'NONE', *, *, #14076, .F. ) ;
#4890=LINE ( 'NONE', #11619, #13113 ) ;
#4903=ORIENTED_EDGE ( 'NONE', *, *, #4547, .T. ) ;
#4904=VERTEX_POINT ( 'NONE', #8880 ) ;
#4905=EDGE_LOOP ( 'NONE', ( #8003, #13256, #10, #7280 ) ) ;
#4916=AXIS2_PLACEMENT_3D ( 'NONE', #12490, #13892, #13821 ) ;
#4986=VECTOR ( 'NONE', #12027, 1000.000000000000000 ) ;
#4997=CARTESIAN_POINT ( 'NONE',  ( 20.00000000000000000, 78.00000000000000000, 25.00000000000000000 ) ) ;
#5005=DIRECTION ( 'NONE',  ( 0.2425356250363328581, -0.9701425001453318764, 0.000000000000000000 ) ) ;
#5013=CYLINDRICAL_SURFACE ( 'NONE', #1214, 2.100000000000000977 ) ;
#5022=VERTEX_POINT ( 'NONE', #2378 ) ;
#5037=EDGE_LOOP ( 'NONE', ( #741, #3661, #11875, #1311 ) ) ;
#5038=LINE ( 'NONE', #2859, #4762 ) ;
#5044=DIRECTION ( 'NONE',  ( -0.000000000000000000, -1.000000000000000000, -0.000000000000000000 ) ) ;
#5053=ORIENTED_EDGE ( 'NONE', *, *, #1983, .F. ) ;
#5056=PLANE ( 'NONE',  #3278 ) ;
#5064=VERTEX_POINT ( 'NONE', #1557 ) ;
#5066=LINE ( 'NONE', #6441, #8059 ) ;
#5079=LINE ( 'NONE', #10794, #11376 ) ;
#5085=ORIENTED_EDGE ( 'NONE', *, *, #4565, .F. ) ;
#5095=ORIENTED_EDGE ( 'NONE', *, *, #11919, .T. ) ;
#5097=DIRECTION ( 'NONE',  ( -0.9701425001453319874, -0.2425356250363328858, 0.000000000000000000 ) ) ;
#5098=VECTOR ( 'NONE', #6261, 1000.000000000000000 ) ;
#5101=EDGE_CURVE ( 'NONE', #5665, #12241, #4718, .T. ) ;
#5102=VERTEX_POINT ( 'NONE', #1716 ) ;
#5117=DIRECTION ( 'NONE',  ( 0.000000000000000000, 0.000000000000000000, -1.000000000000000000 ) ) ;
#5127=AXIS2_PLACEMENT_3D ( 'NONE', #12797, #7307, #12645 ) ;
#5143=LINE ( 'NONE', #10850, #4360 ) ;
#5157=FACE_OUTER_BOUND ( 'NONE', #9297, .T. ) ;
#5159=EDGE_LOOP ( 'NONE', ( #7101, #5437, #11398 ) ) ;
#5163=EDGE_LOOP ( 'NONE', ( #3443, #9031, #9692, #6186 ) ) ;
#5168=ORIENTED_EDGE ( 'NONE', *, *, #5510, .T. ) ;
#5176=CARTESIAN_POINT ( 'NONE',  ( 24.99999999999999289, -4.898587196589414604E-15, 25.00000000000000000 ) ) ;
#5183=VERTEX_POINT ( 'NONE', #5222 ) ;
#5193=DIRECTION ( 'NONE',  ( -1.000000000000000000, 0.000000000000000000, 0.000000000000000000 ) ) ;
#5210=DIRECTION ( 'NONE',  ( -1.000000000000000000, -0.000000000000000000, -0.000000000000000000 ) ) ;
#5213=ORIENTED_EDGE ( 'NONE', *, *, #4236, .T. ) ;
#5222=CARTESIAN_POINT ( 'NONE',  ( 24.99999999999999289, -4.898587196589414604E-15, 25.00000000000000000 ) ) ;
#5244=AXIS2_PLACEMENT_3D ( 'NONE', #4007, #8377, #9333 ) ;
#5246=PLANE ( 'NONE',  #3494 ) ;
#5250=DIRECTION ( 'NONE',  ( 0.000000000000000000, 0.000000000000000000, -1.000000000000000000 ) ) ;
#5269=VERTEX_POINT ( 'NONE', #9613 ) ;
#5270=CARTESIAN_POINT ( 'NONE',  ( 22.00000000000000355, 50.00000000000000000, -25.00000000000000000 ) ) ;
#5283=LINE ( 'NONE', #13055, #8719 ) ;
#5285=EDGE_CURVE ( 'NONE', #12157, #7235, #4890, .T. ) ;
#5289=DIRECTION ( 'NONE',  ( -0.000000000000000000, -1.000000000000000000, -0.000000000000000000 ) ) ;
#5299=CARTESIAN_POINT ( 'NONE',  ( 20.00000000000000000, 27.00000000000000355, 25.00000000000000000 ) ) ;
#5315=CARTESIAN_POINT ( 'NONE',  ( 0.000000000000000000, 0.000000000000000000, -25.00000000000000000 ) ) ;
#5328=VECTOR ( 'NONE', #10815, 1000.000000000000000 ) ;
#5337=VECTOR ( 'NONE', #8683, 1000.000000000000000 ) ;
#5343=SHAPE_REPRESENTATION ( 'Hardened Serrated Safety Wedge', ( #11025 ), #6359 ) ;
#5353=DIRECTION ( 'NONE',  ( -0.000000000000000000, 1.000000000000000000, 0.000000000000000000 ) ) ;
#5359=PLANE ( 'NONE',  #10533 ) ;
#5382=EDGE_CURVE ( 'NONE', #373, #6157, #4818, .T. ) ;
#5384=CYLINDRICAL_SURFACE ( 'NONE', #8128, 2.000000000000001776 ) ;
#5389=ORIENTED_EDGE ( 'NONE', *, *, #1565, .F. ) ;
#5393=ADVANCED_FACE ( 'NONE', ( #294 ), #11694, .T. ) ;
#5394=VECTOR ( 'NONE', #11265, 1000.000000000000000 ) ;
#5395=VERTEX_POINT ( 'NONE', #10527 ) ;
#5408=DIRECTION ( 'NONE',  ( 0.000000000000000000, -0.000000000000000000, 1.000000000000000000 ) ) ;
#5413=EDGE_CURVE ( 'NONE', #337, #4861, #509, .T. ) ;
#5416=DIRECTION ( 'NONE',  ( -0.2425356250363328581, 0.9701425001453318764, 0.000000000000000000 ) ) ;
#5426=STYLED_ITEM ( 'NONE', ( #11213 ), #1042 ) ;
#5437=ORIENTED_EDGE ( 'NONE', *, *, #5285, .T. ) ;
#5441=DIRECTION ( 'NONE',  ( 1.000000000000000000, 0.000000000000000000, 0.000000000000000000 ) ) ;
#5443=DIRECTION ( 'NONE',  ( 0.000000000000000000, 0.000000000000000000, -1.000000000000000000 ) ) ;
#5450=VECTOR ( 'NONE', #11131, 1000.000000000000000 ) ;
#5451=CARTESIAN_POINT ( 'NONE',  ( 22.00000000000000711, 20.00000000000000355, 25.00000000000000000 ) ) ;
#5455=VERTEX_POINT ( 'NONE', #1755 ) ;
#5485=FACE_OUTER_BOUND ( 'NONE', #6269, .T. ) ;
#5510=EDGE_CURVE ( 'NONE', #1722, #9071, #10956, .T. ) ;
#5529=ORIENTED_EDGE ( 'NONE', *, *, #8616, .F. ) ;
#5543=DIRECTION ( 'NONE',  ( 1.000000000000000000, 0.000000000000000000, 0.000000000000000000 ) ) ;
#5548=ORIENTED_EDGE ( 'NONE', *, *, #13094, .T. ) ;
#5549=AXIS2_PLACEMENT_3D ( 'NONE', #5315, #1748, #718 ) ;
#5550=CARTESIAN_POINT ( 'NONE',  ( 54.35294117647056567, -1.411764705882362358, -23.00000000000000000 ) ) ;
#5559=EDGE_CURVE ( 'NONE', #11907, #4680, #10150, .T. ) ;
#5571=FACE_OUTER_BOUND ( 'NONE', #12119, .T. ) ;
#5575=DIRECTION ( 'NONE',  ( -0.2425356250363328581, 0.9701425001453318764, 0.000000000000000000 ) ) ;
#5576=( LENGTH_UNIT ( ) NAMED_UNIT ( * ) SI_UNIT ( .MILLI., .METRE. ) );
#5613=ORIENTED_EDGE ( 'NONE', *, *, #13008, .F. ) ;
#5625=EDGE_LOOP ( 'NONE', ( #10950, #3394, #286, #13456 ) ) ;
#5632=CIRCLE ( 'NONE', #7970, 2.100000000000000977 ) ;
#5639=LINE ( 'NONE', #13913, #13321 ) ;
#5641=VECTOR ( 'NONE', #12730, 1000.000000000000000 ) ;
#5662=CARTESIAN_POINT ( 'NONE',  ( 22.00000000000000000, 78.00000000000000000, 25.00000000000000000 ) ) ;
#5665=VERTEX_POINT ( 'NONE', #11027 ) ;
#5687=VERTEX_POINT ( 'NONE', #10283 ) ;
#5696=DIRECTION ( 'NONE',  ( -1.000000000000000000, -0.000000000000000000, -0.000000000000000000 ) ) ;
#5700=CLOSED_SHELL ( 'NONE', ( #123, #9823, #12280, #8861, #13095, #1809, #8687, #6435, #11113, #5725, #11522, #6285, #3040, #4785, #8898, #4404, #1446, #2997, #736, #14155, #5393, #9502, #6232, #7351, #3280, #9273, #9038, #6847, #8187, #3039, #12190, #5990, #7668, #8107, #11634, #7039, #6891, #1909, #11294, #3789, #14110, #13799, #12065, #11354 ) ) ;
#5707=( NAMED_UNIT ( * ) SI_UNIT ( $, .STERADIAN. ) SOLID_ANGLE_UNIT ( ) );
#5709=ORIENTED_EDGE ( 'NONE', *, *, #2064, .T. ) ;
#5723=ORIENTED_EDGE ( 'NONE', *, *, #2770, .T. ) ;
#5725=ADVANCED_FACE ( 'NONE', ( #273 ), #2765, .F. ) ;
#5733=EDGE_CURVE ( 'NONE', #1722, #5395, #3646, .T. ) ;
#5736=CARTESIAN_POINT ( 'NONE',  ( 0.000000000000000000, 0.000000000000000000, 25.00000000000000000 ) ) ;
#5737=LINE ( 'NONE', #12627, #941 ) ;
#5743=LINE ( 'NONE', #210, #2663 ) ;
#5775=ORIENTED_EDGE ( 'NONE', *, *, #2090, .T. ) ;
#5792=DIRECTION ( 'NONE',  ( 1.000000000000000000, 0.000000000000000000, 0.000000000000000000 ) ) ;
#5818=DIRECTION ( 'NONE',  ( -0.8571673007021134438, 0.000000000000000000, -0.5150380749100522682 ) ) ;
#5824=VERTEX_POINT ( 'NONE', #11761 ) ;
#5830=EDGE_CURVE ( 'NONE', #12564, #14306, #3062, .T. ) ;
#5841=EDGE_LOOP ( 'NONE', ( #6121, #1024, #6748, #13725 ) ) ;
#5911=VECTOR ( 'NONE', #587, 1000.000000000000227 ) ;
#5919=DIRECTION ( 'NONE',  ( 0.000000000000000000, 0.000000000000000000, -1.000000000000000000 ) ) ;
#5952=FACE_OUTER_BOUND ( 'NONE', #2492, .T. ) ;
#5955=DIRECTION ( 'NONE',  ( 1.000000000000000000, 0.000000000000000000, 0.000000000000000000 ) ) ;
#5973=LINE ( 'NONE', #10529, #11912 ) ;
#5981=LINE ( 'NONE', #12580, #11274 ) ;
#5990=ADVANCED_FACE ( 'NONE', ( #12262 ), #9991, .T. ) ;
#6016=CARTESIAN_POINT ( 'NONE',  ( 54.35294117647056567, -1.411764705882362358, 25.00000000000000000 ) ) ;
#6033=CARTESIAN_POINT ( 'NONE',  ( 22.00000000000000000, 78.00000000000000000, -25.00000000000000000 ) ) ;
#6034=VECTOR ( 'NONE', #9493, 1000.000000000000000 ) ;
#6037=CARTESIAN_POINT ( 'NONE',  ( 20.00000000000000000, 78.00000000000000000, 25.00000000000000000 ) ) ;
#6045=VECTOR ( 'NONE', #6052, 1000.000000000000000 ) ;
#6046=DIRECTION ( 'NONE',  ( -0.000000000000000000, -1.000000000000000000, -0.000000000000000000 ) ) ;
#6052=DIRECTION ( 'NONE',  ( 1.000000000000000000, 0.000000000000000000, 0.000000000000000000 ) ) ;
#6059=CARTESIAN_POINT ( 'NONE',  ( 20.00000000000000355, 50.00000000000000000, 25.00000000000000000 ) ) ;
#6066=ORIENTED_EDGE ( 'NONE', *, *, #1647, .F. ) ;
#6075=CARTESIAN_POINT ( 'NONE',  ( 22.00000000000000711, 17.00000000000000000, -25.00000000000000000 ) ) ;
#6078=ORIENTED_EDGE ( 'NONE', *, *, #3298, .T. ) ;
#6086=VECTOR ( 'NONE', #12384, 1000.000000000000000 ) ;
#6099=EDGE_CURVE ( 'NONE', #8027, #4861, #10190, .T. ) ;
#6109=CARTESIAN_POINT ( 'NONE',  ( 22.00000000000000355, 40.00000000000000711, 25.00000000000000000 ) ) ;
#6121=ORIENTED_EDGE ( 'NONE', *, *, #14219, .F. ) ;
#6138=DIRECTION ( 'NONE',  ( 0.000000000000000000, -1.000000000000000000, 0.000000000000000000 ) ) ;
#6156=CARTESIAN_POINT ( 'NONE',  ( 20.00000000000000355, 50.00000000000000000, -25.00000000000000000 ) ) ;
#6157=VERTEX_POINT ( 'NONE', #11889 ) ;
#6161=ORIENTED_EDGE ( 'NONE', *, *, #11383, .T. ) ;
#6162=UNCERTAINTY_MEASURE_WITH_UNIT (LENGTH_MEASURE( 1.000000000000000082E-05 ), #5576, 'distance_accuracy_value', 'NONE');
#6163=CARTESIAN_POINT ( 'NONE',  ( 22.00000000000000355, 40.00000000000000711, 25.00000000000000000 ) ) ;
#6180=ORIENTED_EDGE ( 'NONE', *, *, #8242, .T. ) ;
#6186=ORIENTED_EDGE ( 'NONE', *, *, #7735, .F. ) ;
#6207=ORIENTED_EDGE ( 'NONE', *, *, #12626, .T. ) ;
#6213=FACE_OUTER_BOUND ( 'NONE', #5159, .T. ) ;
#6229=CARTESIAN_POINT ( 'NONE',  ( 20.00000000000000711, 20.00000000000000355, -25.00000000000000000 ) ) ;
#6230=EDGE_CURVE ( 'NONE', #6341, #8772, #7546, .T. ) ;
#6232=ADVANCED_FACE ( 'NONE', ( #13141 ), #5359, .T. ) ;
#6253=AXIS2_PLACEMENT_3D ( 'NONE', #8606, #5097, #9498 ) ;
#6256=ORIENTED_EDGE ( 'NONE', *, *, #9790, .T. ) ;
#6261=DIRECTION ( 'NONE',  ( -0.000000000000000000, -1.000000000000000000, -0.000000000000000000 ) ) ;
#6264=LINE ( 'NONE', #9713, #12799 ) ;
#6269=EDGE_LOOP ( 'NONE', ( #209, #2008, #4493, #3783 ) ) ;
#6277=DIRECTION ( 'NONE',  ( 0.000000000000000000, 0.000000000000000000, -1.000000000000000000 ) ) ;
#6285=ADVANCED_FACE ( 'NONE', ( #892, #5571 ), #12167, .T. ) ;
#6288=VECTOR ( 'NONE', #3883, 1000.000000000000000 ) ;
#6293=FACE_OUTER_BOUND ( 'NONE', #6456, .T. ) ;
#6297=CARTESIAN_POINT ( 'NONE',  ( 20.00000000000000000, 37.00000000000000711, -25.00000000000000000 ) ) ;
#6309=ORIENTED_EDGE ( 'NONE', *, *, #3965, .F. ) ;
#6313=EDGE_LOOP ( 'NONE', ( #12345, #744, #4408, #12438 ) ) ;
#6317=VECTOR ( 'NONE', #2922, 1000.000000000000000 ) ;
#6319=DIRECTION ( 'NONE',  ( -0.000000000000000000, 0.000000000000000000, 1.000000000000000000 ) ) ;
#6327=CIRCLE ( 'NONE', #7260, 2.100000000000000977 ) ;
#6328=EDGE_LOOP ( 'NONE', ( #11727, #13455, #12853, #9143 ) ) ;
#6338=CARTESIAN_POINT ( 'NONE',  ( 20.00000000000000000, 37.00000000000000711, 25.00000000000000000 ) ) ;
#6341=VERTEX_POINT ( 'NONE', #11207 ) ;
#6351=FACE_OUTER_BOUND ( 'NONE', #3913, .T. ) ;
#6359=( GEOMETRIC_REPRESENTATION_CONTEXT ( 3 ) GLOBAL_UNCERTAINTY_ASSIGNED_CONTEXT ( ( #6162 ) ) GLOBAL_UNIT_ASSIGNED_CONTEXT ( ( #5576, #9011, #5707 ) ) REPRESENTATION_CONTEXT ( 'NONE', 'WORKASPACE' ) );
#6360=AXIS2_PLACEMENT_3D ( 'NONE', #3396, #8717, #8855 ) ;
#6371=VECTOR ( 'NONE', #10969, 1000.000000000000114 ) ;
#6378=CARTESIAN_POINT ( 'NONE',  ( 20.00000000000000000, -5.510910596163090344E-15, 25.00000000000000000 ) ) ;
#6392=DIRECTION ( 'NONE',  ( 0.000000000000000000, 0.000000000000000000, 1.000000000000000000 ) ) ;
#6402=ORIENTED_EDGE ( 'NONE', *, *, #6099, .F. ) ;
#6416=CARTESIAN_POINT ( 'NONE',  ( 20.00000000000000000, 80.00000000000000000, -25.00000000000000000 ) ) ;
#6434=LINE ( 'NONE', #6156, #10557 ) ;
#6435=ADVANCED_FACE ( 'NONE', ( #3814 ), #7146, .F. ) ;
#6441=CARTESIAN_POINT ( 'NONE',  ( 20.00000000000000000, 37.00000000000000711, 25.00000000000000000 ) ) ;
#6443=EDGE_CURVE ( 'NONE', #9934, #5064, #5639, .T. ) ;
#6446=CARTESIAN_POINT ( 'NONE',  ( 22.00000000000000000, 60.00000000000000711, 25.00000000000000000 ) ) ;
#6456=EDGE_LOOP ( 'NONE', ( #8538, #12170, #13518, #11251 ) ) ;
#6476=ORIENTED_EDGE ( 'NONE', *, *, #2084, .F. ) ;
#6478=ORIENTED_EDGE ( 'NONE', *, *, #13008, .T. ) ;
#6509=EDGE_CURVE ( 'NONE', #9523, #1217, #11286, .T. ) ;
#6511=DIRECTION ( 'NONE',  ( 0.000000000000000000, 0.000000000000000000, -1.000000000000000000 ) ) ;
#6524=DIRECTION ( 'NONE',  ( 0.000000000000000000, 0.000000000000000000, 1.000000000000000000 ) ) ;
#6578=VERTEX_POINT ( 'NONE', #1975 ) ;
#6579=FACE_OUTER_BOUND ( 'NONE', #905, .T. ) ;
#6582=CARTESIAN_POINT ( 'NONE',  ( 22.00000000000000000, 80.00000000000000000, 25.00000000000000000 ) ) ;
#6584=VECTOR ( 'NONE', #1248, 1000.000000000000000 ) ;
#6597=DIRECTION ( 'NONE',  ( 0.000000000000000000, -0.000000000000000000, 1.000000000000000000 ) ) ;
#6606=CARTESIAN_POINT ( 'NONE',  ( 20.00000000000000000, -5.510910596163090344E-15, 25.00000000000000000 ) ) ;
#6621=LINE ( 'NONE', #10063, #2071 ) ;
#6637=DIRECTION ( 'NONE',  ( -1.000000000000000000, 0.000000000000000000, 0.000000000000000000 ) ) ;
#6642=ORIENTED_EDGE ( 'NONE', *, *, #11882, .F. ) ;
#6647=ORIENTED_EDGE ( 'NONE', *, *, #14097, .F. ) ;
#6652=DIRECTION ( 'NONE',  ( 1.000000000000000000, 0.000000000000000000, 0.000000000000000000 ) ) ;
#6654=PLANE ( 'NONE',  #6694 ) ;
#6689=CARTESIAN_POINT ( 'NONE',  ( 20.00000000000000355, 17.00000000000000000, -25.00000000000000000 ) ) ;
#6694=AXIS2_PLACEMENT_3D ( 'NONE', #3235, #4277, #12152 ) ;
#6723=ORIENTED_EDGE ( 'NONE', *, *, #3619, .T. ) ;
#6725=DIRECTION ( 'NONE',  ( 0.000000000000000000, -0.000000000000000000, 1.000000000000000000 ) ) ;
#6728=LINE ( 'NONE', #6582, #10080 ) ;
#6738=CARTESIAN_POINT ( 'NONE',  ( 20.00000000000000000, 70.00000000000000000, 25.00000000000000000 ) ) ;
#6748=ORIENTED_EDGE ( 'NONE', *, *, #10141, .T. ) ;
#6756=EDGE_CURVE ( 'NONE', #1060, #8772, #2324, .T. ) ;
#6762=VERTEX_POINT ( 'NONE', #9039 ) ;
#6767=MANIFOLD_SOLID_BREP ( 'AdvancedHole1', #5700 ) ;
#6768=ORIENTED_EDGE ( 'NONE', *, *, #14124, .F. ) ;
#6775=CARTESIAN_POINT ( 'NONE',  ( 20.00000000000000355, 40.00000000000000711, 25.00000000000000000 ) ) ;
#6776=EDGE_CURVE ( 'NONE', #9291, #3573, #3288, .T. ) ;
#6795=LINE ( 'NONE', #12368, #5394 ) ;
#6804=EDGE_CURVE ( 'NONE', #9644, #13416, #3648, .T. ) ;
#6836=DIRECTION ( 'NONE',  ( -0.000000000000000000, 1.000000000000000000, -0.000000000000000000 ) ) ;
#6841=DIRECTION ( 'NONE',  ( 0.000000000000000000, 0.000000000000000000, -1.000000000000000000 ) ) ;
#6847=ADVANCED_FACE ( 'NONE', ( #9262 ), #13746, .T. ) ;
#6856=FILL_AREA_STYLE ('',( #4669 ) ) ;
#6868=CARTESIAN_POINT ( 'NONE',  ( 22.00000000000000355, 40.00000000000000711, 25.00000000000000000 ) ) ;
#6891=ADVANCED_FACE ( 'NONE', ( #789 ), #5246, .F. ) ;
#6909=ORIENTED_EDGE ( 'NONE', *, *, #2055, .T. ) ;
#6918=FACE_OUTER_BOUND ( 'NONE', #2754, .T. ) ;
#6936=ORIENTED_EDGE ( 'NONE', *, *, #6804, .F. ) ;
#6947=AXIS2_PLACEMENT_3D ( 'NONE', #6868, #13107, #12000 ) ;
#6967=LINE ( 'NONE', #3698, #730 ) ;
#6977=ORIENTED_EDGE ( 'NONE', *, *, #311, .T. ) ;
#6987=DIRECTION ( 'NONE',  ( 0.000000000000000000, 0.000000000000000000, -1.000000000000000000 ) ) ;
#7027=ORIENTED_EDGE ( 'NONE', *, *, #5413, .T. ) ;
#7028=DIRECTION ( 'NONE',  ( -0.000000000000000000, -0.000000000000000000, -1.000000000000000000 ) ) ;
#7039=ADVANCED_FACE ( 'NONE', ( #8679 ), #5384, .T. ) ;
#7046=ORIENTED_EDGE ( 'NONE', *, *, #2680, .F. ) ;
#7061=DIRECTION ( 'NONE',  ( -1.000000000000000000, 0.000000000000000000, 0.000000000000000000 ) ) ;
#7069=EDGE_LOOP ( 'NONE', ( #10727, #12418, #11155, #14032 ) ) ;
#7070=EDGE_CURVE ( 'NONE', #6578, #13498, #6621, .T. ) ;
#7074=CARTESIAN_POINT ( 'NONE',  ( 57.35294117647057277, -1.411764705882362358, -23.00000000000000000 ) ) ;
#7075=LINE ( 'NONE', #4686, #258 ) ;
#7095=ORIENTED_EDGE ( 'NONE', *, *, #14443, .F. ) ;
#7101=ORIENTED_EDGE ( 'NONE', *, *, #3923, .F. ) ;
#7106=CARTESIAN_POINT ( 'NONE',  ( 54.35294117647056567, -1.411764705882362358, -25.00000000000000000 ) ) ;
#7132=( LENGTH_UNIT ( ) NAMED_UNIT ( * ) SI_UNIT ( .MILLI., .METRE. ) );
#7138=CARTESIAN_POINT ( 'NONE',  ( 53.99999999999997868, -1.347111479062091166E-15, 25.00000000000000000 ) ) ;
#7146=PLANE ( 'NONE',  #5127 ) ;
#7149=DIRECTION ( 'NONE',  ( 0.000000000000000000, 0.000000000000000000, -1.000000000000000000 ) ) ;
#7181=VECTOR ( 'NONE', #4543, 1000.000000000000000 ) ;
#7188=CARTESIAN_POINT ( 'NONE',  ( 28.00000000000000355, 29.99999999999999645, -25.00000000000000000 ) ) ;
#7233=CARTESIAN_POINT ( 'NONE',  ( 20.00000000000000000, 5.000000000000000000, -25.00000000000000000 ) ) ;
#7235=VERTEX_POINT ( 'NONE', #3773 ) ;
#7254=CARTESIAN_POINT ( 'NONE',  ( 30.10000000000000497, 29.99999999999999645, -6.999999999999992006 ) ) ;
#7257=ORIENTED_EDGE ( 'NONE', *, *, #2805, .F. ) ;
#7260=AXIS2_PLACEMENT_3D ( 'NONE', #7188, #11895, #12927 ) ;
#7269=ORIENTED_EDGE ( 'NONE', *, *, #5285, .F. ) ;
#7277=AXIS2_PLACEMENT_3D ( 'NONE', #864, #5117, #5193 ) ;
#7278=DIRECTION ( 'NONE',  ( -0.000000000000000000, 1.000000000000000000, 0.000000000000000000 ) ) ;
#7280=ORIENTED_EDGE ( 'NONE', *, *, #11548, .F. ) ;
#7302=DIRECTION ( 'NONE',  ( -0.000000000000000000, -0.000000000000000000, -1.000000000000000000 ) ) ;
#7307=DIRECTION ( 'NONE',  ( 1.000000000000000000, 0.000000000000000000, 0.000000000000000000 ) ) ;
#7315=ORIENTED_EDGE ( 'NONE', *, *, #5733, .F. ) ;
#7316=EDGE_CURVE ( 'NONE', #181, #2621, #8444, .T. ) ;
#7318=EDGE_CURVE ( 'NONE', #14168, #12241, #2978, .T. ) ;
#7323=CARTESIAN_POINT ( 'NONE',  ( 20.00000000000000355, 30.00000000000000711, -25.00000000000000000 ) ) ;
#7347=CARTESIAN_POINT ( 'NONE',  ( 40.00000000000000711, 80.00000000000000000, 25.00000000000000000 ) ) ;
#7348=EDGE_CURVE ( 'NONE', #1645, #1073, #12761, .T. ) ;
#7351=ADVANCED_FACE ( 'NONE', ( #5157 ), #9619, .T. ) ;
#7353=CARTESIAN_POINT ( 'NONE',  ( 30.10000000000000497, 29.99999999999999645, -25.00000000000000000 ) ) ;
#7362=DIRECTION ( 'NONE',  ( 0.000000000000000000, -0.000000000000000000, -1.000000000000000000 ) ) ;
#7366=PLANE ( 'NONE',  #6253 ) ;
#7398=CARTESIAN_POINT ( 'NONE',  ( 60.00000000000000000, -6.123233995736768255E-16, 25.00000000000000000 ) ) ;
#7418=CARTESIAN_POINT ( 'NONE',  ( 19.99999999999999645, 57.00000000000000000, -25.00000000000000000 ) ) ;
#7425=ORIENTED_EDGE ( 'NONE', *, *, #8014, .T. ) ;
#7432=VECTOR ( 'NONE', #6836, 1000.000000000000000 ) ;
#7433=EDGE_CURVE ( 'NONE', #721, #1722, #13215, .T. ) ;
#7541=DIRECTION ( 'NONE',  ( -0.2425356250363328581, 0.9701425001453318764, 0.000000000000000000 ) ) ;
#7542=AXIS2_PLACEMENT_3D ( 'NONE', #11395, #9122, #12365 ) ;
#7543=CARTESIAN_POINT ( 'NONE',  ( 22.00000000000000000, 67.00000000000000000, 25.00000000000000000 ) ) ;
#7546=LINE ( 'NONE', #8653, #11702 ) ;
#7605=LINE ( 'NONE', #10246, #6086 ) ;
#7607=PRODUCT_DEFINITION_CONTEXT ( 'detailed design', #4309, 'design' ) ;
#7609=CARTESIAN_POINT ( 'NONE',  ( 20.00000000000000000, 37.00000000000000711, -25.00000000000000000 ) ) ;
#7610=DIRECTION ( 'NONE',  ( 0.000000000000000000, -1.000000000000000000, 0.000000000000000000 ) ) ;
#7611=CARTESIAN_POINT ( 'NONE',  ( 0.000000000000000000, 0.000000000000000000, -25.00000000000000000 ) ) ;
#7618=LINE ( 'NONE', #9832, #166 ) ;
#7624=AXIS2_PLACEMENT_3D ( 'NONE', #1169, #3169, #14429 ) ;
#7634=ORIENTED_EDGE ( 'NONE', *, *, #8828, .T. ) ;
#7643=CARTESIAN_POINT ( 'NONE',  ( 56.99999999999997868, -1.031959805901694782E-15, -23.00000000000000000 ) ) ;
#7668=ADVANCED_FACE ( 'NONE', ( #7985 ), #12460, .T. ) ;
#7669=ORIENTED_EDGE ( 'NONE', *, *, #14316, .T. ) ;
#7680=CARTESIAN_POINT ( 'NONE',  ( 40.00000000000000711, 80.00000000000000000, 25.00000000000000000 ) ) ;
#7692=VECTOR ( 'NONE', #13194, 1000.000000000000000 ) ;
#7700=ORIENTED_EDGE ( 'NONE', *, *, #5510, .F. ) ;
#7705=VERTEX_POINT ( 'NONE', #12589 ) ;
#7730=SURFACE_STYLE_USAGE ( .BOTH. , #10214 ) ;
#7735=EDGE_CURVE ( 'NONE', #10580, #6578, #3837, .T. ) ;
#7743=ORIENTED_EDGE ( 'NONE', *, *, #14366, .F. ) ;
#7785=DIRECTION ( 'NONE',  ( -0.000000000000000000, 1.000000000000000000, 0.000000000000000000 ) ) ;
#7794=EDGE_LOOP ( 'NONE', ( #895, #6256, #8576, #11738 ) ) ;
#7811=EDGE_CURVE ( 'NONE', #4126, #1525, #752, .T. ) ;
#7831=DIRECTION ( 'NONE',  ( 0.000000000000000000, -1.000000000000000000, 0.000000000000000000 ) ) ;
#7901=VERTEX_POINT ( 'NONE', #11 ) ;
#7922=CARTESIAN_POINT ( 'NONE',  ( 22.00000000000000355, 27.00000000000000355, 25.00000000000000000 ) ) ;
#7931=ORIENTED_EDGE ( 'NONE', *, *, #5101, .T. ) ;
#7943=DIRECTION ( 'NONE',  ( 0.000000000000000000, 0.000000000000000000, -1.000000000000000000 ) ) ;
#7960=DIRECTION ( 'NONE',  ( -1.000000000000000000, -0.000000000000000000, -0.000000000000000000 ) ) ;
#7970=AXIS2_PLACEMENT_3D ( 'NONE', #297, #11554, #12369 ) ;
#7985=FACE_OUTER_BOUND ( 'NONE', #5841, .T. ) ;
#7989=VECTOR ( 'NONE', #4413, 1000.000000000000000 ) ;
#7996=DIRECTION ( 'NONE',  ( -1.000000000000000000, -0.000000000000000000, -0.000000000000000000 ) ) ;
#8001=VERTEX_POINT ( 'NONE', #3173 ) ;
#8003=ORIENTED_EDGE ( 'NONE', *, *, #9321, .F. ) ;
#8005=ORIENTED_EDGE ( 'NONE', *, *, #1007, .F. ) ;
#8014=EDGE_CURVE ( 'NONE', #11907, #1563, #9269, .T. ) ;
#8019=ORIENTED_EDGE ( 'NONE', *, *, #4531, .T. ) ;
#8027=VERTEX_POINT ( 'NONE', #4882 ) ;
#8059=VECTOR ( 'NONE', #10914, 1000.000000000000000 ) ;
#8103=DIRECTION ( 'NONE',  ( 0.000000000000000000, 0.000000000000000000, -1.000000000000000000 ) ) ;
#8107=ADVANCED_FACE ( 'NONE', ( #8997 ), #3457, .T. ) ;
#8115=CARTESIAN_POINT ( 'NONE',  ( 22.00000000000000711, 17.00000000000000000, 25.00000000000000000 ) ) ;
#8128=AXIS2_PLACEMENT_3D ( 'NONE', #5662, #2098, #12980 ) ;
#8138=ORIENTED_EDGE ( 'NONE', *, *, #936, .F. ) ;
#8147=VECTOR ( 'NONE', #5044, 1000.000000000000000 ) ;
#8187=ADVANCED_FACE ( 'NONE', ( #10741 ), #2933, .T. ) ;
#8204=CARTESIAN_POINT ( 'NONE',  ( 28.00000000000000355, 29.99999999999999645, -6.999999999999992006 ) ) ;
#8206=VECTOR ( 'NONE', #12629, 1000.000000000000000 ) ;
#8242=EDGE_CURVE ( 'NONE', #9976, #14165, #10878, .T. ) ;
#8255=LINE ( 'NONE', #12727, #11710 ) ;
#8273=EDGE_CURVE ( 'NONE', #13731, #1368, #9574, .T. ) ;
#8289=DIRECTION ( 'NONE',  ( -0.000000000000000000, -0.000000000000000000, -1.000000000000000000 ) ) ;
#8291=EDGE_LOOP ( 'NONE', ( #538, #13836, #5529, #14320 ) ) ;
#8295=EDGE_LOOP ( 'NONE', ( #3967, #4767, #6180, #329 ) ) ;
#8299=ORIENTED_EDGE ( 'NONE', *, *, #14217, .F. ) ;
#8302=( NAMED_UNIT ( * ) SI_UNIT ( $, .STERADIAN. ) SOLID_ANGLE_UNIT ( ) );
#8336=DIRECTION ( 'NONE',  ( -1.000000000000000000, -0.000000000000000000, -0.000000000000000000 ) ) ;
#8337=EDGE_CURVE ( 'NONE', #5102, #5269, #2314, .T. ) ;
#8348=PRODUCT_DEFINITION_SHAPE ( 'NONE', 'NONE',  #9274 ) ;
#8352=CARTESIAN_POINT ( 'NONE',  ( 22.00000000000000000, 57.00000000000000000, 25.00000000000000000 ) ) ;
#8363=DIRECTION ( 'NONE',  ( -1.000000000000000000, 0.000000000000000000, 0.000000000000000000 ) ) ;
#8364=ORIENTED_EDGE ( 'NONE', *, *, #14279, .F. ) ;
#8375=ORIENTED_EDGE ( 'NONE', *, *, #8242, .F. ) ;
#8377=DIRECTION ( 'NONE',  ( 0.000000000000000000, -1.000000000000000000, 0.000000000000000000 ) ) ;
#8383=DIRECTION ( 'NONE',  ( -0.000000000000000000, 0.000000000000000000, -1.000000000000000000 ) ) ;
#8388=CARTESIAN_POINT ( 'NONE',  ( 20.00000000000000711, 20.00000000000000355, 25.00000000000000000 ) ) ;
#8396=VECTOR ( 'NONE', #14060, 1000.000000000000000 ) ;
#8415=CARTESIAN_POINT ( 'NONE',  ( 20.00000000000000000, -5.510910596163090344E-15, 25.00000000000000000 ) ) ;
#8427=EDGE_CURVE ( 'NONE', #9564, #6762, #336, .T. ) ;
#8443=DIRECTION ( 'NONE',  ( 1.000000000000000000, 1.224646799147353454E-16, 0.000000000000000000 ) ) ;
#8444=LINE ( 'NONE', #2907, #13980 ) ;
#8467=ORIENTED_EDGE ( 'NONE', *, *, #11383, .F. ) ;
#8474=VECTOR ( 'NONE', #8998, 1000.000000000000000 ) ;
#8482=CARTESIAN_POINT ( 'NONE',  ( 36.99999999999999289, 80.00000000000000000, 25.00000000000000000 ) ) ;
#8496=CARTESIAN_POINT ( 'NONE',  ( 20.00000000000000000, -5.510910596163090344E-15, 25.00000000000000000 ) ) ;
#8508=UNCERTAINTY_MEASURE_WITH_UNIT (LENGTH_MEASURE( 1.000000000000000082E-05 ), #7132, 'distance_accuracy_value', 'NONE');
#8512=DIRECTION ( 'NONE',  ( 0.000000000000000000, 0.000000000000000000, -1.000000000000000000 ) ) ;
#8520=ORIENTED_EDGE ( 'NONE', *, *, #6756, .T. ) ;
#8537=LINE ( 'NONE', #2994, #2776 ) ;
#8538=ORIENTED_EDGE ( 'NONE', *, *, #9196, .F. ) ;
#8544=EDGE_CURVE ( 'NONE', #9291, #1178, #5079, .T. ) ;
#8576=ORIENTED_EDGE ( 'NONE', *, *, #2998, .F. ) ;
#8581=VECTOR ( 'NONE', #3337, 1000.000000000000114 ) ;
#8586=CARTESIAN_POINT ( 'NONE',  ( 53.99999999999997868, -1.347111479062091166E-15, 25.00000000000000000 ) ) ;
#8606=CARTESIAN_POINT ( 'NONE',  ( 40.00000000000000711, 80.00000000000000000, 25.00000000000000000 ) ) ;
#8615=ORIENTED_EDGE ( 'NONE', *, *, #8273, .F. ) ;
#8616=EDGE_CURVE ( 'NONE', #5269, #14306, #9622, .T. ) ;
#8617=EDGE_CURVE ( 'NONE', #14306, #6762, #7618, .T. ) ;
#8619=AXIS2_PLACEMENT_3D ( 'NONE', #3718, #2613, #7362 ) ;
#8650=LINE ( 'NONE', #10913, #9361 ) ;
#8651=DIRECTION ( 'NONE',  ( -0.000000000000000000, 1.000000000000000000, -0.000000000000000000 ) ) ;
#8653=CARTESIAN_POINT ( 'NONE',  ( 20.00000000000000000, -5.510910596163090344E-15, 25.00000000000000000 ) ) ;
#8675=LINE ( 'NONE', #12052, #10477 ) ;
#8679=FACE_OUTER_BOUND ( 'NONE', #5163, .T. ) ;
#8683=DIRECTION ( 'NONE',  ( 0.000000000000000000, 0.000000000000000000, -1.000000000000000000 ) ) ;
#8687=ADVANCED_FACE ( 'NONE', ( #3127 ), #975, .F. ) ;
#8696=CARTESIAN_POINT ( 'NONE',  ( 28.00000000000000355, 29.99999999999999645, -6.999999999999992006 ) ) ;
#8709=ORIENTED_EDGE ( 'NONE', *, *, #7070, .F. ) ;
#8717=DIRECTION ( 'NONE',  ( 0.000000000000000000, -1.000000000000000000, 0.000000000000000000 ) ) ;
#8719=VECTOR ( 'NONE', #14224, 1000.000000000000000 ) ;
#8748=FACE_OUTER_BOUND ( 'NONE', #8295, .T. ) ;
#8772=VERTEX_POINT ( 'NONE', #9115 ) ;
#8774=VECTOR ( 'NONE', #762, 1000.000000000000000 ) ;
#8777=LINE ( 'NONE', #874, #7692 ) ;
#8803=SURFACE_SIDE_STYLE ('',( #8945 ) ) ;
#8808=ORIENTED_EDGE ( 'NONE', *, *, #1889, .F. ) ;
#8815=LINE ( 'NONE', #4163, #8835 ) ;
#8826=ORIENTED_EDGE ( 'NONE', *, *, #14279, .T. ) ;
#8828=EDGE_CURVE ( 'NONE', #13043, #5183, #6264, .T. ) ;
#8834=CARTESIAN_POINT ( 'NONE',  ( 20.00000000000000355, 30.00000000000000711, 25.00000000000000000 ) ) ;
#8835=VECTOR ( 'NONE', #13088, 1000.000000000000000 ) ;
#8846=DIRECTION ( 'NONE',  ( -0.2425356250363328581, 0.9701425001453318764, 0.000000000000000000 ) ) ;
#8855=DIRECTION ( 'NONE',  ( 0.000000000000000000, -0.000000000000000000, -1.000000000000000000 ) ) ;
#8861=ADVANCED_FACE ( 'NONE', ( #14120 ), #9776, .T. ) ;
#8869=ORIENTED_EDGE ( 'NONE', *, *, #10881, .T. ) ;
#8880=CARTESIAN_POINT ( 'NONE',  ( 22.00000000000000355, 47.00000000000000000, -25.00000000000000000 ) ) ;
#8898=ADVANCED_FACE ( 'NONE', ( #12781 ), #7366, .F. ) ;
#8918=LINE ( 'NONE', #5550, #6371 ) ;
#8935=AXIS2_PLACEMENT_3D ( 'NONE', #8496, #10766, #11941 ) ;
#8944=EDGE_CURVE ( 'NONE', #5102, #12564, #13022, .T. ) ;
#8945=SURFACE_STYLE_FILL_AREA ( #28 ) ;
#8946=EDGE_CURVE ( 'NONE', #5022, #4126, #1815, .T. ) ;
#8959=EDGE_LOOP ( 'NONE', ( #7269, #13474, #8869 ) ) ;
#8981=CARTESIAN_POINT ( 'NONE',  ( 22.00000000000000000, 78.00000000000000000, 25.00000000000000000 ) ) ;
#8991=CARTESIAN_POINT ( 'NONE',  ( 20.00000000000000000, 47.00000000000000000, -25.00000000000000000 ) ) ;
#8997=FACE_OUTER_BOUND ( 'NONE', #13568, .T. ) ;
#8998=DIRECTION ( 'NONE',  ( -0.000000000000000000, 1.000000000000000000, -0.000000000000000000 ) ) ;
#9009=ORIENTED_EDGE ( 'NONE', *, *, #2646, .F. ) ;
#9011=( NAMED_UNIT ( * ) PLANE_ANGLE_UNIT ( ) SI_UNIT ( $, .RADIAN. ) );
#9030=AXIS2_PLACEMENT_3D ( 'NONE', #6606, #12107, #5443 ) ;
#9031=ORIENTED_EDGE ( 'NONE', *, *, #12048, .F. ) ;
#9038=ADVANCED_FACE ( 'NONE', ( #6351 ), #2037, .T. ) ;
#9039=CARTESIAN_POINT ( 'NONE',  ( 33.99999999999998579, 80.00000000000000000, 25.00000000000000000 ) ) ;
#9040=CARTESIAN_POINT ( 'NONE',  ( 19.99999999999999645, 57.00000000000000000, 25.00000000000000000 ) ) ;
#9045=VECTOR ( 'NONE', #8289, 1000.000000000000000 ) ;
#9067=CIRCLE ( 'NONE', #10230, 2.000000000000001776 ) ;
#9071=VERTEX_POINT ( 'NONE', #13242 ) ;
#9078=( NAMED_UNIT ( * ) PLANE_ANGLE_UNIT ( ) SI_UNIT ( $, .RADIAN. ) );
#9079=ORIENTED_EDGE ( 'NONE', *, *, #12048, .T. ) ;
#9102=ORIENTED_EDGE ( 'NONE', *, *, #10141, .F. ) ;
#9115=CARTESIAN_POINT ( 'NONE',  ( 20.00000000000000355, 40.00000000000000711, 25.00000000000000000 ) ) ;
#9122=DIRECTION ( 'NONE',  ( -0.000000000000000000, -0.000000000000000000, -1.000000000000000000 ) ) ;
#9129=LINE ( 'NONE', #4755, #223 ) ;
#9143=ORIENTED_EDGE ( 'NONE', *, *, #4681, .T. ) ;
#9176=EDGE_LOOP ( 'NONE', ( #3135, #12375, #8019, #8005 ) ) ;
#9189=EDGE_CURVE ( 'NONE', #181, #777, #66, .T. ) ;
#9190=ORIENTED_EDGE ( 'NONE', *, *, #429, .F. ) ;
#9196=EDGE_CURVE ( 'NONE', #5064, #2621, #11173, .T. ) ;
#9201=ORIENTED_EDGE ( 'NONE', *, *, #13931, .F. ) ;
#9211=CARTESIAN_POINT ( 'NONE',  ( 20.00000000000000355, 50.00000000000000000, 25.00000000000000000 ) ) ;
#9225=EDGE_LOOP ( 'NONE', ( #1634, #211, #6647, #9860 ) ) ;
#9259=VERTEX_POINT ( 'NONE', #9040 ) ;
#9262=FACE_OUTER_BOUND ( 'NONE', #12128, .T. ) ;
#9269=LINE ( 'NONE', #355, #434 ) ;
#9273=ADVANCED_FACE ( 'NONE', ( #3506 ), #11321, .T. ) ;
#9274=PRODUCT_DEFINITION ( 'UNKNOWN', '', #12014, #7607 ) ;
#9291=VERTEX_POINT ( 'NONE', #13609 ) ;
#9297=EDGE_LOOP ( 'NONE', ( #8138, #634, #9642, #13328 ) ) ;
#9321=EDGE_CURVE ( 'NONE', #5022, #13659, #2694, .T. ) ;
#9327=EDGE_CURVE ( 'NONE', #6578, #9071, #9067, .T. ) ;
#9333=DIRECTION ( 'NONE',  ( 0.000000000000000000, -0.000000000000000000, -1.000000000000000000 ) ) ;
#9336=( GEOMETRIC_REPRESENTATION_CONTEXT ( 3 ) GLOBAL_UNCERTAINTY_ASSIGNED_CONTEXT ( ( #8508 ) ) GLOBAL_UNIT_ASSIGNED_CONTEXT ( ( #7132, #11680, #8302 ) ) REPRESENTATION_CONTEXT ( 'NONE', 'WORKASPACE' ) );
#9346=EDGE_CURVE ( 'NONE', #1507, #651, #3946, .T. ) ;
#9353=DIRECTION ( 'NONE',  ( 0.000000000000000000, 0.000000000000000000, -1.000000000000000000 ) ) ;
#9357=VECTOR ( 'NONE', #177, 1000.000000000000000 ) ;
#9358=CARTESIAN_POINT ( 'NONE',  ( 20.00000000000000000, -5.510910596163090344E-15, 25.00000000000000000 ) ) ;
#9361=VECTOR ( 'NONE', #9899, 1000.000000000000000 ) ;
#9363=EDGE_CURVE ( 'NONE', #8001, #1060, #1661, .T. ) ;
#9372=AXIS2_PLACEMENT_3D ( 'NONE', #9358, #2638, #7149 ) ;
#9373=EDGE_CURVE ( 'NONE', #3543, #721, #11604, .T. ) ;
#9413=VECTOR ( 'NONE', #5543, 1000.000000000000000 ) ;
#9417=CARTESIAN_POINT ( 'NONE',  ( 28.00000000000000355, 29.99999999999999645, -25.00000000000000000 ) ) ;
#9432=CARTESIAN_POINT ( 'NONE',  ( 22.00000000000000355, 30.00000000000000711, -25.00000000000000000 ) ) ;
#9454=DIRECTION ( 'NONE',  ( 0.000000000000000000, 0.000000000000000000, -1.000000000000000000 ) ) ;
#9472=CARTESIAN_POINT ( 'NONE',  ( 28.00000000000000355, 29.99999999999999645, -25.00000000000000000 ) ) ;
#9493=DIRECTION ( 'NONE',  ( -0.000000000000000000, -1.000000000000000000, -0.000000000000000000 ) ) ;
#9498=DIRECTION ( 'NONE',  ( 0.2425356250363328581, -0.9701425001453318764, 0.000000000000000000 ) ) ;
#9502=ADVANCED_FACE ( 'NONE', ( #8748 ), #1883, .T. ) ;
#9508=FACE_OUTER_BOUND ( 'NONE', #12909, .T. ) ;
#9521=EDGE_LOOP ( 'NONE', ( #1675, #5709, #12715, #4043 ) ) ;
#9523=VERTEX_POINT ( 'NONE', #4103 ) ;
#9534=UNCERTAINTY_MEASURE_WITH_UNIT (LENGTH_MEASURE( 1.000000000000000082E-05 ), #12320, 'distance_accuracy_value', 'NONE');
#9535=EDGE_CURVE ( 'NONE', #9644, #1073, #8537, .T. ) ;
#9555=ORIENTED_EDGE ( 'NONE', *, *, #7318, .F. ) ;
#9564=VERTEX_POINT ( 'NONE', #11366 ) ;
#9568=DIRECTION ( 'NONE',  ( -0.9701425001453319874, -0.2425356250363328858, 0.000000000000000000 ) ) ;
#9574=LINE ( 'NONE', #1887, #890 ) ;
#9577=LINE ( 'NONE', #10602, #12960 ) ;
#9581=LINE ( 'NONE', #1680, #4672 ) ;
#9588=VECTOR ( 'NONE', #4753, 1000.000000000000000 ) ;
#9599=DIRECTION ( 'NONE',  ( 1.000000000000000000, 0.000000000000000000, 0.000000000000000000 ) ) ;
#9613=CARTESIAN_POINT ( 'NONE',  ( 53.99999999999997868, -1.324077043022348342E-15, 23.00000000000000000 ) ) ;
#9619=PLANE ( 'NONE',  #2757 ) ;
#9622=LINE ( 'NONE', #14107, #8581 ) ;
#9641=DIRECTION ( 'NONE',  ( 0.000000000000000000, -0.000000000000000000, 1.000000000000000000 ) ) ;
#9642=ORIENTED_EDGE ( 'NONE', *, *, #6099, .T. ) ;
#9644=VERTEX_POINT ( 'NONE', #6689 ) ;
#9654=LINE ( 'NONE', #10607, #8396 ) ;
#9667=VECTOR ( 'NONE', #9744, 1000.000000000000000 ) ;
#9670=DIRECTION ( 'NONE',  ( 1.000000000000000000, 0.000000000000000000, 0.000000000000000000 ) ) ;
#9692=ORIENTED_EDGE ( 'NONE', *, *, #9327, .F. ) ;
#9694=ORIENTED_EDGE ( 'NONE', *, *, #2805, .T. ) ;
#9713=CARTESIAN_POINT ( 'NONE',  ( 24.99999999999999289, -4.898587196589414604E-15, 25.00000000000000000 ) ) ;
#9718=CARTESIAN_POINT ( 'NONE',  ( 60.00000000000000000, -6.123233995736768255E-16, -25.00000000000000000 ) ) ;
#9733=DIRECTION ( 'NONE',  ( -0.000000000000000000, 1.000000000000000000, -0.000000000000000000 ) ) ;
#9736=VECTOR ( 'NONE', #8512, 1000.000000000000000 ) ;
#9743=VECTOR ( 'NONE', #5416, 1000.000000000000114 ) ;
#9744=DIRECTION ( 'NONE',  ( -0.000000000000000000, 1.000000000000000000, -0.000000000000000000 ) ) ;
#9775=AXIS2_PLACEMENT_3D ( 'NONE', #12056, #719, #9641 ) ;
#9776=PLANE ( 'NONE',  #5549 ) ;
#9780=VECTOR ( 'NONE', #7996, 1000.000000000000000 ) ;
#9782=ORIENTED_EDGE ( 'NONE', *, *, #4236, .F. ) ;
#9790=EDGE_CURVE ( 'NONE', #6157, #7901, #10491, .T. ) ;
#9795=APPLICATION_CONTEXT ( 'automotive_design' ) ;
#9808=PLANE ( 'NONE',  #7624 ) ;
#9811=ORIENTED_EDGE ( 'NONE', *, *, #1743, .F. ) ;
#9823=ADVANCED_FACE ( 'NONE', ( #553 ), #5013, .F. ) ;
#9832=CARTESIAN_POINT ( 'NONE',  ( 33.99999999999998579, 80.00000000000000000, 25.00000000000000000 ) ) ;
#9860=ORIENTED_EDGE ( 'NONE', *, *, #10392, .T. ) ;
#9892=CARTESIAN_POINT ( 'NONE',  ( 20.00000000000000000, 5.000000000000000000, 25.00000000000000000 ) ) ;
#9895=AXIS2_PLACEMENT_3D ( 'NONE', #1852, #755, #7541 ) ;
#9899=DIRECTION ( 'NONE',  ( -0.000000000000000000, 1.000000000000000000, -0.000000000000000000 ) ) ;
#9917=ORIENTED_EDGE ( 'NONE', *, *, #14217, .T. ) ;
#9920=DIRECTION ( 'NONE',  ( 1.000000000000000000, 0.000000000000000000, 0.000000000000000000 ) ) ;
#9926=CARTESIAN_POINT ( 'NONE',  ( 20.00000000000000711, 20.00000000000000355, 25.00000000000000000 ) ) ;
#9934=VERTEX_POINT ( 'NONE', #6446 ) ;
#9949=ORIENTED_EDGE ( 'NONE', *, *, #13537, .T. ) ;
#9950=VECTOR ( 'NONE', #101, 1000.000000000000000 ) ;
#9954=CARTESIAN_POINT ( 'NONE',  ( 57.35294117647057277, -1.411764705882362358, 25.00000000000000000 ) ) ;
#9957=CARTESIAN_POINT ( 'NONE',  ( 20.00000000000000000, -5.510910596163090344E-15, 25.00000000000000000 ) ) ;
#9964=FACE_OUTER_BOUND ( 'NONE', #3131, .T. ) ;
#9976=VERTEX_POINT ( 'NONE', #10990 ) ;
#9988=CARTESIAN_POINT ( 'NONE',  ( 20.00000000000000000, 27.00000000000000355, -25.00000000000000000 ) ) ;
#9990=VECTOR ( 'NONE', #2527, 1000.000000000000114 ) ;
#9991=PLANE ( 'NONE',  #12868 ) ;
#10002=ORIENTED_EDGE ( 'NONE', *, *, #742, .T. ) ;
#10008=VECTOR ( 'NONE', #10433, 1000.000000000000000 ) ;
#10009=DIRECTION ( 'NONE',  ( -0.000000000000000000, -0.000000000000000000, -1.000000000000000000 ) ) ;
#10019=CARTESIAN_POINT ( 'NONE',  ( 20.00000000000000000, 80.00000000000000000, 25.00000000000000000 ) ) ;
#10029=ORIENTED_EDGE ( 'NONE', *, *, #2016, .T. ) ;
#10031=PLANE ( 'NONE',  #6360 ) ;
#10050=DIRECTION ( 'NONE',  ( 0.000000000000000000, -0.000000000000000000, 1.000000000000000000 ) ) ;
#10062=VERTEX_POINT ( 'NONE', #4825 ) ;
#10063=CARTESIAN_POINT ( 'NONE',  ( 20.00000000000000000, -5.510910596163090344E-15, -25.00000000000000000 ) ) ;
#10080=VECTOR ( 'NONE', #11057, 1000.000000000000000 ) ;
#10097=FACE_OUTER_BOUND ( 'NONE', #6313, .T. ) ;
#10100=FACE_OUTER_BOUND ( 'NONE', #1246, .T. ) ;
#10120=SHAPE_REPRESENTATION_RELATIONSHIP ( 'NONE' , 'NONE' ,  #5343, #1042 ) ;
#10141=EDGE_CURVE ( 'NONE', #9934, #12581, #1685, .T. ) ;
#10150=LINE ( 'NONE', #2256, #10973 ) ;
#10180=ORIENTED_EDGE ( 'NONE', *, *, #14076, .T. ) ;
#10190=LINE ( 'NONE', #2377, #9357 ) ;
#10214=SURFACE_SIDE_STYLE ('',( #1290 ) ) ;
#10215=CARTESIAN_POINT ( 'NONE',  ( 20.00000000000000000, 37.00000000000000711, 25.00000000000000000 ) ) ;
#10225=DIRECTION ( 'NONE',  ( 0.000000000000000000, 0.000000000000000000, -1.000000000000000000 ) ) ;
#10226=ORIENTED_EDGE ( 'NONE', *, *, #1270, .F. ) ;
#10230=AXIS2_PLACEMENT_3D ( 'NONE', #6033, #8383, #7061 ) ;
#10246=CARTESIAN_POINT ( 'NONE',  ( 33.99999999999998579, 80.00000000000000000, -23.00000000000000000 ) ) ;
#10254=COLOUR_RGB ( '', 0.40784314, 0.44705882, 0.49803922) ;
#10258=VECTOR ( 'NONE', #14197, 1000.000000000000000 ) ;
#10264=LINE ( 'NONE', #14461, #9780 ) ;
#10269=ORIENTED_EDGE ( 'NONE', *, *, #11159, .F. ) ;
#10283=CARTESIAN_POINT ( 'NONE',  ( 22.00000000000000000, 80.00000000000000000, 25.00000000000000000 ) ) ;
#10286=DIRECTION ( 'NONE',  ( -0.2425356250363328581, 0.9701425001453318764, 0.000000000000000000 ) ) ;
#10315=PLANE ( 'NONE',  #10785 ) ;
#10321=ORIENTED_EDGE ( 'NONE', *, *, #13458, .T. ) ;
#10322=ORIENTED_EDGE ( 'NONE', *, *, #1007, .T. ) ;
#10335=CARTESIAN_POINT ( 'NONE',  ( 20.00000000000000355, 17.00000000000000000, 25.00000000000000000 ) ) ;
#10380=CARTESIAN_POINT ( 'NONE',  ( 19.99999999999999645, 67.00000000000000000, -25.00000000000000000 ) ) ;
#10392=EDGE_CURVE ( 'NONE', #12770, #9644, #5737, .T. ) ;
#10397=ORIENTED_EDGE ( 'NONE', *, *, #3162, .T. ) ;
#10406=CARTESIAN_POINT ( 'NONE',  ( 20.00000000000000355, 50.00000000000000000, -25.00000000000000000 ) ) ;
#10419=CARTESIAN_POINT ( 'NONE',  ( 33.99999999999998579, 80.00000000000000000, 23.00000000000000000 ) ) ;
#10424=ORIENTED_EDGE ( 'NONE', *, *, #1743, .T. ) ;
#10426=CARTESIAN_POINT ( 'NONE',  ( 53.99999999999997868, -1.324077043022348342E-15, -25.00000000000000000 ) ) ;
#10433=DIRECTION ( 'NONE',  ( -0.000000000000000000, 1.000000000000000000, -0.000000000000000000 ) ) ;
#10444=ORIENTED_EDGE ( 'NONE', *, *, #2084, .T. ) ;
#10445=CARTESIAN_POINT ( 'NONE',  ( 22.00000000000000711, 20.00000000000000355, 25.00000000000000000 ) ) ;
#10448=DIRECTION ( 'NONE',  ( -0.000000000000000000, 1.000000000000000000, -0.000000000000000000 ) ) ;
#10477=VECTOR ( 'NONE', #2093, 1000.000000000000000 ) ;
#10486=FACE_OUTER_BOUND ( 'NONE', #3265, .T. ) ;
#10491=LINE ( 'NONE', #1639, #3481 ) ;
#10505=FACE_OUTER_BOUND ( 'NONE', #14463, .T. ) ;
#10511=VECTOR ( 'NONE', #11923, 1000.000000000000000 ) ;
#10527=CARTESIAN_POINT ( 'NONE',  ( 33.99999999999998579, 80.00000000000000000, -23.00000000000000000 ) ) ;
#10529=CARTESIAN_POINT ( 'NONE',  ( 20.00000000000000711, 20.00000000000000355, -25.00000000000000000 ) ) ;
#10531=CARTESIAN_POINT ( 'NONE',  ( 20.00000000000000000, -5.510910596163090344E-15, 25.00000000000000000 ) ) ;
#10533=AXIS2_PLACEMENT_3D ( 'NONE', #2287, #4212, #6597 ) ;
#10546=ORIENTED_EDGE ( 'NONE', *, *, #9535, .F. ) ;
#10549=AXIS2_PLACEMENT_3D ( 'NONE', #14201, #2867, #13036 ) ;
#10550=ORIENTED_EDGE ( 'NONE', *, *, #742, .F. ) ;
#10556=ORIENTED_EDGE ( 'NONE', *, *, #13127, .T. ) ;
#10557=VECTOR ( 'NONE', #5210, 1000.000000000000000 ) ;
#10580=VERTEX_POINT ( 'NONE', #6037 ) ;
#10599=VECTOR ( 'NONE', #6511, 1000.000000000000000 ) ;
#10602=CARTESIAN_POINT ( 'NONE',  ( 20.00000000000000000, -5.510910596163090344E-15, 25.00000000000000000 ) ) ;
#10607=CARTESIAN_POINT ( 'NONE',  ( 30.10000000000000497, 29.99999999999999645, -25.00000000000000000 ) ) ;
#10613=PLANE ( 'NONE',  #10549 ) ;
#10631=ORIENTED_EDGE ( 'NONE', *, *, #239, .F. ) ;
#10633=CARTESIAN_POINT ( 'NONE',  ( 20.00000000000000000, -5.510910596163090344E-15, -25.00000000000000000 ) ) ;
#10649=ORIENTED_EDGE ( 'NONE', *, *, #9363, .T. ) ;
#10666=DIRECTION ( 'NONE',  ( -1.000000000000000000, 0.000000000000000000, 0.000000000000000000 ) ) ;
#10684=CARTESIAN_POINT ( 'NONE',  ( 22.00000000000000000, 60.00000000000000711, 25.00000000000000000 ) ) ;
#10711=AXIS2_PLACEMENT_3D ( 'NONE', #9417, #11681, #10666 ) ;
#10715=LINE ( 'NONE', #1793, #9743 ) ;
#10717=ORIENTED_EDGE ( 'NONE', *, *, #2680, .T. ) ;
#10722=ORIENTED_EDGE ( 'NONE', *, *, #2258, .F. ) ;
#10727=ORIENTED_EDGE ( 'NONE', *, *, #7348, .F. ) ;
#10728=ORIENTED_EDGE ( 'NONE', *, *, #7433, .T. ) ;
#10738=DIRECTION ( 'NONE',  ( 0.7071067811865483499, 0.7071067811865467956, 0.000000000000000000 ) ) ;
#10741=FACE_OUTER_BOUND ( 'NONE', #1313, .T. ) ;
#10742=EDGE_CURVE ( 'NONE', #9259, #3170, #3100, .T. ) ;
#10745=ORIENTED_EDGE ( 'NONE', *, *, #14097, .T. ) ;
#10766=DIRECTION ( 'NONE',  ( 1.000000000000000000, 0.000000000000000000, 0.000000000000000000 ) ) ;
#10774=VECTOR ( 'NONE', #8443, 1000.000000000000000 ) ;
#10777=DIRECTION ( 'NONE',  ( -0.000000000000000000, -1.000000000000000000, -0.000000000000000000 ) ) ;
#10778=VECTOR ( 'NONE', #407, 1000.000000000000000 ) ;
#10785=AXIS2_PLACEMENT_3D ( 'NONE', #9211, #6138, #12511 ) ;
#10794=CARTESIAN_POINT ( 'NONE',  ( 60.00000000000000000, -6.123233995736768255E-16, 25.00000000000000000 ) ) ;
#10809=VECTOR ( 'NONE', #6392, 1000.000000000000000 ) ;
#10811=DIRECTION ( 'NONE',  ( 1.000000000000000000, 0.000000000000000000, 0.000000000000000000 ) ) ;
#10815=DIRECTION ( 'NONE',  ( 0.000000000000000000, 0.000000000000000000, -1.000000000000000000 ) ) ;
#10817=VERTEX_POINT ( 'NONE', #8991 ) ;
#10820=VECTOR ( 'NONE', #11049, 1000.000000000000000 ) ;
#10824=ORIENTED_EDGE ( 'NONE', *, *, #5101, .F. ) ;
#10832=FACE_OUTER_BOUND ( 'NONE', #6328, .T. ) ;
#10837=CARTESIAN_POINT ( 'NONE',  ( 20.00000000000000355, 40.00000000000000711, -25.00000000000000000 ) ) ;
#10850=CARTESIAN_POINT ( 'NONE',  ( 22.00000000000000000, 60.00000000000000711, 25.00000000000000000 ) ) ;
#10865=EDGE_LOOP ( 'NONE', ( #1001, #3263, #8299, #10550 ) ) ;
#10872=PLANE ( 'NONE',  #3538 ) ;
#10878=LINE ( 'NONE', #8388, #5337 ) ;
#10881=EDGE_CURVE ( 'NONE', #3193, #7235, #5632, .T. ) ;
#10895=ORIENTED_EDGE ( 'NONE', *, *, #9790, .F. ) ;
#10904=ORIENTED_EDGE ( 'NONE', *, *, #13277, .T. ) ;
#10907=FACE_OUTER_BOUND ( 'NONE', #1388, .T. ) ;
#10913=CARTESIAN_POINT ( 'NONE',  ( 22.00000000000000355, 50.00000000000000000, 25.00000000000000000 ) ) ;
#10914=DIRECTION ( 'NONE',  ( 1.000000000000000000, 0.000000000000000000, 0.000000000000000000 ) ) ;
#10950=ORIENTED_EDGE ( 'NONE', *, *, #1429, .F. ) ;
#10956=LINE ( 'NONE', #6416, #10511 ) ;
#10964=CARTESIAN_POINT ( 'NONE',  ( 20.00000000000000000, 70.00000000000000000, -25.00000000000000000 ) ) ;
#10969=DIRECTION ( 'NONE',  ( -0.2425356250363328581, 0.9701425001453318764, 0.000000000000000000 ) ) ;
#10973=VECTOR ( 'NONE', #7943, 1000.000000000000000 ) ;
#10974=LINE ( 'NONE', #14430, #6584 ) ;
#10977=VERTEX_POINT ( 'NONE', #4037 ) ;
#10990=CARTESIAN_POINT ( 'NONE',  ( 20.00000000000000711, 20.00000000000000355, 25.00000000000000000 ) ) ;
#10993=ORIENTED_EDGE ( 'NONE', *, *, #5559, .T. ) ;
#11005=EDGE_CURVE ( 'NONE', #13731, #9976, #11853, .T. ) ;
#11008=CARTESIAN_POINT ( 'NONE',  ( 20.00000000000000000, 27.00000000000000355, -25.00000000000000000 ) ) ;
#11017=AXIS2_PLACEMENT_3D ( 'NONE', #8696, #10009, #6637 ) ;
#11025=AXIS2_PLACEMENT_3D ( 'NONE', #167, #6524, #5441 ) ;
#11027=CARTESIAN_POINT ( 'NONE',  ( 60.00000000000000000, -6.123233995736768255E-16, -25.00000000000000000 ) ) ;
#11044=LINE ( 'NONE', #14278, #11325 ) ;
#11049=DIRECTION ( 'NONE',  ( -1.000000000000000000, -0.000000000000000000, -0.000000000000000000 ) ) ;
#11052=CIRCLE ( 'NONE', #3588, 2.000000000000001776 ) ;
#11057=DIRECTION ( 'NONE',  ( -0.000000000000000000, -0.000000000000000000, 1.000000000000000000 ) ) ;
#11072=PLANE ( 'NONE',  #157 ) ;
#11113=ADVANCED_FACE ( 'NONE', ( #4689 ), #298, .F. ) ;
#11131=DIRECTION ( 'NONE',  ( -0.7071067811865467956, 0.7071067811865483499, -0.000000000000000000 ) ) ;
#11144=SURFACE_STYLE_USAGE ( .BOTH. , #8803 ) ;
#11148=LINE ( 'NONE', #7922, #12704 ) ;
#11155=ORIENTED_EDGE ( 'NONE', *, *, #72, .T. ) ;
#11159=EDGE_CURVE ( 'NONE', #13731, #4830, #8255, .T. ) ;
#11173=LINE ( 'NONE', #1153, #2760 ) ;
#11200=DIRECTION ( 'NONE',  ( 0.000000000000000000, 0.000000000000000000, -1.000000000000000000 ) ) ;
#11201=VECTOR ( 'NONE', #9353, 1000.000000000000000 ) ;
#11207=CARTESIAN_POINT ( 'NONE',  ( 20.00000000000000000, 47.00000000000000000, 25.00000000000000000 ) ) ;
#11213=PRESENTATION_STYLE_ASSIGNMENT (( #11144 ) ) ;
#11214=AXIS2_PLACEMENT_3D ( 'NONE', #10445, #1596, #2707 ) ;
#11251=ORIENTED_EDGE ( 'NONE', *, *, #7316, .T. ) ;
#11265=DIRECTION ( 'NONE',  ( -1.000000000000000000, -0.000000000000000000, -0.000000000000000000 ) ) ;
#11270=LINE ( 'NONE', #2275, #13384 ) ;
#11274=VECTOR ( 'NONE', #5696, 1000.000000000000000 ) ;
#11278=CARTESIAN_POINT ( 'NONE',  ( 20.00000000000000000, 70.00000000000000000, 25.00000000000000000 ) ) ;
#11284=LINE ( 'NONE', #12165, #9950 ) ;
#11286=LINE ( 'NONE', #1600, #6045 ) ;
#11294=ADVANCED_FACE ( 'NONE', ( #1977 ), #10613, .F. ) ;
#11316=CARTESIAN_POINT ( 'NONE',  ( 25.90000000000000213, 29.99999999999999645, -25.00000000000000000 ) ) ;
#11321=PLANE ( 'NONE',  #1127 ) ;
#11325=VECTOR ( 'NONE', #809, 1000.000000000000000 ) ;
#11354=ADVANCED_FACE ( 'NONE', ( #6213 ), #13608, .F. ) ;
#11366=CARTESIAN_POINT ( 'NONE',  ( 53.99999999999997868, -1.084202172485504434E-15, 25.00000000000000000 ) ) ;
#11376=VECTOR ( 'NONE', #2981, 1000.000000000000000 ) ;
#11383=EDGE_CURVE ( 'NONE', #8027, #13659, #1229, .T. ) ;
#11395=CARTESIAN_POINT ( 'NONE',  ( 28.00000000000000355, 29.99999999999999645, -6.999999999999992006 ) ) ;
#11398=ORIENTED_EDGE ( 'NONE', *, *, #13931, .T. ) ;
#11402=DIRECTION ( 'NONE',  ( -1.000000000000000000, -0.000000000000000000, -0.000000000000000000 ) ) ;
#11410=DIRECTION ( 'NONE',  ( -1.000000000000000000, -0.000000000000000000, -0.000000000000000000 ) ) ;
#11419=ORIENTED_EDGE ( 'NONE', *, *, #11005, .T. ) ;
#11430=DIRECTION ( 'NONE',  ( -0.9701425001453319874, -0.2425356250363328858, 0.000000000000000000 ) ) ;
#11448=AXIS2_PLACEMENT_3D ( 'NONE', #5736, #4671, #1582 ) ;
#11459=DIRECTION ( 'NONE',  ( 0.000000000000000000, 0.000000000000000000, -1.000000000000000000 ) ) ;
#11503=AXIS2_PLACEMENT_3D ( 'NONE', #14453, #10050, #3552 ) ;
#11514=AXIS2_PLACEMENT_3D ( 'NONE', #882, #5353, #13203 ) ;
#11522=ADVANCED_FACE ( 'NONE', ( #6918 ), #1361, .F. ) ;
#11532=CARTESIAN_POINT ( 'NONE',  ( 20.00000000000000000, 47.00000000000000000, 25.00000000000000000 ) ) ;
#11548=EDGE_CURVE ( 'NONE', #13659, #4373, #2470, .T. ) ;
#11549=ORIENTED_EDGE ( 'NONE', *, *, #2998, .T. ) ;
#11554=DIRECTION ( 'NONE',  ( -0.000000000000000000, -0.000000000000000000, -1.000000000000000000 ) ) ;
#11563=ORIENTED_EDGE ( 'NONE', *, *, #9373, .F. ) ;
#11583=DIRECTION ( 'NONE',  ( -0.000000000000000000, -0.000000000000000000, -1.000000000000000000 ) ) ;
#11604=LINE ( 'NONE', #2846, #678 ) ;
#11610=CARTESIAN_POINT ( 'NONE',  ( 36.99999999999999289, 80.00000000000000000, 23.00000000000000000 ) ) ;
#11617=ORIENTED_EDGE ( 'NONE', *, *, #14366, .T. ) ;
#11619=CARTESIAN_POINT ( 'NONE',  ( 25.90000000000000213, 29.99999999999999645, -6.999999999999992006 ) ) ;
#11634=ADVANCED_FACE ( 'NONE', ( #2930 ), #576, .F. ) ;
#11664=DIRECTION ( 'NONE',  ( -0.000000000000000000, -1.000000000000000000, -0.000000000000000000 ) ) ;
#11665=CARTESIAN_POINT ( 'NONE',  ( 20.00000000000000355, 17.00000000000000000, 25.00000000000000000 ) ) ;
#11670=CARTESIAN_POINT ( 'NONE',  ( 22.00000000000000355, 27.00000000000000355, 25.00000000000000000 ) ) ;
#11671=ORIENTED_EDGE ( 'NONE', *, *, #2079, .F. ) ;
#11680=( NAMED_UNIT ( * ) PLANE_ANGLE_UNIT ( ) SI_UNIT ( $, .RADIAN. ) );
#11681=DIRECTION ( 'NONE',  ( -0.000000000000000000, -0.000000000000000000, -1.000000000000000000 ) ) ;
#11694=PLANE ( 'NONE',  #11214 ) ;
#11695=DIRECTION ( 'NONE',  ( -1.000000000000000000, -1.224646799147353454E-16, 0.000000000000000000 ) ) ;
#11696=DIRECTION ( 'NONE',  ( -1.000000000000000000, -0.000000000000000000, -0.000000000000000000 ) ) ;
#11702=VECTOR ( 'NONE', #5289, 1000.000000000000000 ) ;
#11709=LINE ( 'NONE', #5270, #11992 ) ;
#11710=VECTOR ( 'NONE', #8103, 1000.000000000000000 ) ;
#11727=ORIENTED_EDGE ( 'NONE', *, *, #6776, .F. ) ;
#11738=ORIENTED_EDGE ( 'NONE', *, *, #3162, .F. ) ;
#11740=CARTESIAN_POINT ( 'NONE',  ( 40.00000000000000711, 80.00000000000000000, -25.00000000000000000 ) ) ;
#11755=DIRECTION ( 'NONE',  ( 0.000000000000000000, -0.000000000000000000, 1.000000000000000000 ) ) ;
#11761=CARTESIAN_POINT ( 'NONE',  ( 22.00000000000000355, 50.00000000000000000, -25.00000000000000000 ) ) ;
#11781=LINE ( 'NONE', #12724, #2327 ) ;
#11829=EDGE_CURVE ( 'NONE', #10062, #4904, #6967, .T. ) ;
#11830=CARTESIAN_POINT ( 'NONE',  ( 22.00000000000000355, 37.00000000000000711, -25.00000000000000000 ) ) ;
#11844=EDGE_LOOP ( 'NONE', ( #10269, #2577, #2009, #13284 ) ) ;
#11849=EDGE_LOOP ( 'NONE', ( #1120, #234, #3445, #6642 ) ) ;
#11851=CARTESIAN_POINT ( 'NONE',  ( 20.00000000000000000, -5.510910596163090344E-15, 25.00000000000000000 ) ) ;
#11853=LINE ( 'NONE', #10531, #2600 ) ;
#11859=VECTOR ( 'NONE', #5919, 1000.000000000000000 ) ;
#11864=ORIENTED_EDGE ( 'NONE', *, *, #12501, .T. ) ;
#11875=ORIENTED_EDGE ( 'NONE', *, *, #4070, .T. ) ;
#11882=EDGE_CURVE ( 'NONE', #7705, #373, #1796, .T. ) ;
#11889=CARTESIAN_POINT ( 'NONE',  ( 36.99999999999999289, 80.00000000000000000, -23.00000000000000000 ) ) ;
#11895=DIRECTION ( 'NONE',  ( -0.000000000000000000, -0.000000000000000000, -1.000000000000000000 ) ) ;
#11899=ORIENTED_EDGE ( 'NONE', *, *, #7316, .F. ) ;
#11902=VECTOR ( 'NONE', #10286, 1000.000000000000114 ) ;
#11907=VERTEX_POINT ( 'NONE', #1723 ) ;
#11912=VECTOR ( 'NONE', #11696, 1000.000000000000000 ) ;
#11919=EDGE_CURVE ( 'NONE', #651, #1507, #6327, .T. ) ;
#11923=DIRECTION ( 'NONE',  ( -1.000000000000000000, -0.000000000000000000, -0.000000000000000000 ) ) ;
#11935=EDGE_LOOP ( 'NONE', ( #10631, #92, #10180, #6768 ) ) ;
#11941=DIRECTION ( 'NONE',  ( 0.000000000000000000, 0.000000000000000000, -1.000000000000000000 ) ) ;
#11969=LINE ( 'NONE', #8586, #10809 ) ;
#11992=VECTOR ( 'NONE', #9733, 1000.000000000000000 ) ;
#11994=ORIENTED_EDGE ( 'NONE', *, *, #11882, .T. ) ;
#12000=DIRECTION ( 'NONE',  ( -0.000000000000000000, 0.000000000000000000, 1.000000000000000000 ) ) ;
#12014=PRODUCT_DEFINITION_FORMATION_WITH_SPECIFIED_SOURCE ( 'ANY', '', #1709, .NOT_KNOWN. ) ;
#12027=DIRECTION ( 'NONE',  ( -0.000000000000000000, -1.000000000000000000, -0.000000000000000000 ) ) ;
#12043=ORIENTED_EDGE ( 'NONE', *, *, #7811, .T. ) ;
#12048=EDGE_CURVE ( 'NONE', #9071, #5687, #6728, .T. ) ;
#12052=CARTESIAN_POINT ( 'NONE',  ( 22.00000000000000355, 50.00000000000000000, 25.00000000000000000 ) ) ;
#12056=CARTESIAN_POINT ( 'NONE',  ( 20.00000000000000000, 47.00000000000000000, 25.00000000000000000 ) ) ;
#12065=ADVANCED_FACE ( 'NONE', ( #10100 ), #14431, .F. ) ;
#12088=LINE ( 'NONE', #6378, #12242 ) ;
#12107=DIRECTION ( 'NONE',  ( 1.000000000000000000, 0.000000000000000000, 0.000000000000000000 ) ) ;
#12114=LINE ( 'NONE', #9988, #12202 ) ;
#12119=EDGE_LOOP ( 'NONE', ( #13176, #11563, #9917, #6936, #2735, #13380, #6909, #3806, #6723, #7027, #10424, #2570, #12043, #6207, #7669, #3324, #8826, #10321, #14327, #4888, #14176, #5723, #13306, #11899, #12292, #5548, #10904, #8709, #3364, #7700 ) ) ;
#12128=EDGE_LOOP ( 'NONE', ( #13307, #8520, #10322, #12597 ) ) ;
#12146=ORIENTED_EDGE ( 'NONE', *, *, #161, .T. ) ;
#12152=DIRECTION ( 'NONE',  ( -0.000000000000000000, 0.000000000000000000, 1.000000000000000000 ) ) ;
#12157=VERTEX_POINT ( 'NONE', #521 ) ;
#12165=CARTESIAN_POINT ( 'NONE',  ( 22.00000000000000355, 37.00000000000000711, 25.00000000000000000 ) ) ;
#12167=PLANE ( 'NONE',  #4244 ) ;
#12170=ORIENTED_EDGE ( 'NONE', *, *, #2090, .F. ) ;
#12186=VECTOR ( 'NONE', #8336, 1000.000000000000000 ) ;
#12190=ADVANCED_FACE ( 'NONE', ( #13847 ), #10315, .T. ) ;
#12194=VECTOR ( 'NONE', #12212, 1000.000000000000000 ) ;
#12201=CARTESIAN_POINT ( 'NONE',  ( 22.00000000000000355, 50.00000000000000000, 25.00000000000000000 ) ) ;
#12202=VECTOR ( 'NONE', #9920, 1000.000000000000000 ) ;
#12209=PRESENTATION_STYLE_ASSIGNMENT (( #7730 ) ) ;
#12212=DIRECTION ( 'NONE',  ( -1.000000000000000000, -0.000000000000000000, -0.000000000000000000 ) ) ;
#12220=DIRECTION ( 'NONE',  ( -1.000000000000000000, 0.000000000000000000, 0.000000000000000000 ) ) ;
#12241=VERTEX_POINT ( 'NONE', #13700 ) ;
#12242=VECTOR ( 'NONE', #10777, 1000.000000000000000 ) ;
#12245=DIRECTION ( 'NONE',  ( 0.000000000000000000, -0.000000000000000000, -1.000000000000000000 ) ) ;
#12262=FACE_OUTER_BOUND ( 'NONE', #5625, .T. ) ;
#12280=ADVANCED_FACE ( 'NONE', ( #10832 ), #806, .F. ) ;
#12292=ORIENTED_EDGE ( 'NONE', *, *, #9189, .T. ) ;
#12301=DIRECTION ( 'NONE',  ( 1.000000000000000000, 0.000000000000000000, 0.000000000000000000 ) ) ;
#12311=ORIENTED_EDGE ( 'NONE', *, *, #7070, .T. ) ;
#12320=( LENGTH_UNIT ( ) NAMED_UNIT ( * ) SI_UNIT ( .MILLI., .METRE. ) );
#12345=ORIENTED_EDGE ( 'NONE', *, *, #11829, .F. ) ;
#12365=DIRECTION ( 'NONE',  ( -1.000000000000000000, 0.000000000000000000, 0.000000000000000000 ) ) ;
#12368=CARTESIAN_POINT ( 'NONE',  ( 20.00000000000000711, 20.00000000000000355, 25.00000000000000000 ) ) ;
#12369=DIRECTION ( 'NONE',  ( -1.000000000000000000, 0.000000000000000000, 0.000000000000000000 ) ) ;
#12375=ORIENTED_EDGE ( 'NONE', *, *, #2085, .T. ) ;
#12384=DIRECTION ( 'NONE',  ( 1.000000000000000000, 0.000000000000000000, 0.000000000000000000 ) ) ;
#12395=DIRECTION ( 'NONE',  ( 0.000000000000000000, 0.000000000000000000, -1.000000000000000000 ) ) ;
#12418=ORIENTED_EDGE ( 'NONE', *, *, #13211, .T. ) ;
#12438=ORIENTED_EDGE ( 'NONE', *, *, #13458, .F. ) ;
#12446=( GEOMETRIC_REPRESENTATION_CONTEXT ( 3 ) GLOBAL_UNCERTAINTY_ASSIGNED_CONTEXT ( ( #9534 ) ) GLOBAL_UNIT_ASSIGNED_CONTEXT ( ( #12320, #9078, #1122 ) ) REPRESENTATION_CONTEXT ( 'NONE', 'WORKASPACE' ) );
#12455=LINE ( 'NONE', #228, #11859 ) ;
#12460=PLANE ( 'NONE',  #4634 ) ;
#12486=ORIENTED_EDGE ( 'NONE', *, *, #8427, .T. ) ;
#12489=ORIENTED_EDGE ( 'NONE', *, *, #9373, .T. ) ;
#12490=CARTESIAN_POINT ( 'NONE',  ( 20.00000000000000000, -5.510910596163090344E-15, 25.00000000000000000 ) ) ;
#12492=CARTESIAN_POINT ( 'NONE',  ( 57.35294117647057277, -1.411764705882362358, 25.00000000000000000 ) ) ;
#12501=EDGE_CURVE ( 'NONE', #5269, #9564, #3725, .T. ) ;
#12511=DIRECTION ( 'NONE',  ( 0.000000000000000000, -0.000000000000000000, -1.000000000000000000 ) ) ;
#12523=ORIENTED_EDGE ( 'NONE', *, *, #2016, .F. ) ;
#12551=DIRECTION ( 'NONE',  ( 0.000000000000000000, 0.000000000000000000, 1.000000000000000000 ) ) ;
#12564=VERTEX_POINT ( 'NONE', #11610 ) ;
#12580=CARTESIAN_POINT ( 'NONE',  ( 20.00000000000000000, 70.00000000000000000, -25.00000000000000000 ) ) ;
#12581=VERTEX_POINT ( 'NONE', #12866 ) ;
#12589=CARTESIAN_POINT ( 'NONE',  ( 53.99999999999997868, -1.324077043022348342E-15, -23.00000000000000000 ) ) ;
#12597=ORIENTED_EDGE ( 'NONE', *, *, #14316, .F. ) ;
#12605=VECTOR ( 'NONE', #1527, 1000.000000000000114 ) ;
#12609=ORIENTED_EDGE ( 'NONE', *, *, #2258, .T. ) ;
#12617=VECTOR ( 'NONE', #12551, 1000.000000000000000 ) ;
#12622=LINE ( 'NONE', #11532, #3919 ) ;
#12626=EDGE_CURVE ( 'NONE', #1525, #1016, #10974, .T. ) ;
#12627=CARTESIAN_POINT ( 'NONE',  ( 20.00000000000000355, 17.00000000000000000, 25.00000000000000000 ) ) ;
#12629=DIRECTION ( 'NONE',  ( 0.000000000000000000, 0.000000000000000000, 1.000000000000000000 ) ) ;
#12645=DIRECTION ( 'NONE',  ( 0.000000000000000000, 0.000000000000000000, -1.000000000000000000 ) ) ;
#12673=EDGE_CURVE ( 'NONE', #13416, #13043, #11270, .T. ) ;
#12689=VECTOR ( 'NONE', #13308, 1000.000000000000000 ) ;
#12695=LINE ( 'NONE', #485, #10778 ) ;
#12704=VECTOR ( 'NONE', #12395, 1000.000000000000000 ) ;
#12715=ORIENTED_EDGE ( 'NONE', *, *, #9346, .T. ) ;
#12719=ORIENTED_EDGE ( 'NONE', *, *, #9346, .F. ) ;
#12724=CARTESIAN_POINT ( 'NONE',  ( 20.00000000000000000, -5.510910596163090344E-15, 25.00000000000000000 ) ) ;
#12727=CARTESIAN_POINT ( 'NONE',  ( 20.00000000000000000, 27.00000000000000355, 25.00000000000000000 ) ) ;
#12730=DIRECTION ( 'NONE',  ( 0.000000000000000000, 0.000000000000000000, -1.000000000000000000 ) ) ;
#12739=CARTESIAN_POINT ( 'NONE',  ( 20.00000000000000355, 30.00000000000000711, -25.00000000000000000 ) ) ;
#12761=LINE ( 'NONE', #4150, #871 ) ;
#12770=VERTEX_POINT ( 'NONE', #10335 ) ;
#12781=FACE_OUTER_BOUND ( 'NONE', #2453, .T. ) ;
#12797=CARTESIAN_POINT ( 'NONE',  ( 20.00000000000000000, -5.510910596163090344E-15, 25.00000000000000000 ) ) ;
#12799=VECTOR ( 'NONE', #654, 1000.000000000000000 ) ;
#12811=ORIENTED_EDGE ( 'NONE', *, *, #9363, .F. ) ;
#12846=VECTOR ( 'NONE', #197, 1000.000000000000000 ) ;
#12853=ORIENTED_EDGE ( 'NONE', *, *, #305, .T. ) ;
#12854=CARTESIAN_POINT ( 'NONE',  ( 24.99999999999999289, -4.898587196589414604E-15, 25.00000000000000000 ) ) ;
#12866=CARTESIAN_POINT ( 'NONE',  ( 22.00000000000000000, 60.00000000000000711, -25.00000000000000000 ) ) ;
#12868=AXIS2_PLACEMENT_3D ( 'NONE', #3347, #7785, #4521 ) ;
#12907=EDGE_CURVE ( 'NONE', #5824, #14008, #6434, .T. ) ;
#12908=LINE ( 'NONE', #13135, #9667 ) ;
#12909=EDGE_LOOP ( 'NONE', ( #12489, #4845, #11994, #10397, #3746, #7046, #14428, #1768, #13655, #11864, #10722, #10002 ) ) ;
#12927=DIRECTION ( 'NONE',  ( -1.000000000000000000, 0.000000000000000000, 0.000000000000000000 ) ) ;
#12933=CARTESIAN_POINT ( 'NONE',  ( 22.00000000000000355, 27.00000000000000355, -25.00000000000000000 ) ) ;
#12934=ORIENTED_EDGE ( 'NONE', *, *, #4029, .F. ) ;
#12960=VECTOR ( 'NONE', #6046, 1000.000000000000000 ) ;
#12980=DIRECTION ( 'NONE',  ( -1.000000000000000000, 0.000000000000000000, 0.000000000000000000 ) ) ;
#12984=CARTESIAN_POINT ( 'NONE',  ( 33.99999999999998579, 80.00000000000000000, -25.00000000000000000 ) ) ;
#12990=PLANE ( 'NONE',  #9895 ) ;
#13008=EDGE_CURVE ( 'NONE', #1563, #13498, #97, .T. ) ;
#13022=LINE ( 'NONE', #1886, #426 ) ;
#13031=LINE ( 'NONE', #1974, #2100 ) ;
#13036=DIRECTION ( 'NONE',  ( -1.000000000000000000, 0.000000000000000000, -0.000000000000000000 ) ) ;
#13043=VERTEX_POINT ( 'NONE', #9892 ) ;
#13047=DIRECTION ( 'NONE',  ( 0.000000000000000000, 0.000000000000000000, -1.000000000000000000 ) ) ;
#13055=CARTESIAN_POINT ( 'NONE',  ( 20.00000000000000355, 50.00000000000000000, 25.00000000000000000 ) ) ;
#13073=DIRECTION ( 'NONE',  ( -1.000000000000000000, 0.000000000000000000, -0.000000000000000000 ) ) ;
#13088=DIRECTION ( 'NONE',  ( -0.000000000000000000, -0.000000000000000000, -1.000000000000000000 ) ) ;
#13094=EDGE_CURVE ( 'NONE', #777, #4680, #4284, .T. ) ;
#13095=ADVANCED_FACE ( 'NONE', ( #9964 ), #10031, .F. ) ;
#13103=AXIS2_PLACEMENT_3D ( 'NONE', #9954, #3308, #8846 ) ;
#13107=DIRECTION ( 'NONE',  ( -1.000000000000000000, 0.000000000000000000, -0.000000000000000000 ) ) ;
#13113=VECTOR ( 'NONE', #5818, 1000.000000000000000 ) ;
#13123=PLANE ( 'NONE',  #8935 ) ;
#13127=EDGE_CURVE ( 'NONE', #435, #13438, #4351, .T. ) ;
#13131=VECTOR ( 'NONE', #6652, 1000.000000000000000 ) ;
#13135=CARTESIAN_POINT ( 'NONE',  ( 22.00000000000000711, 20.00000000000000355, -25.00000000000000000 ) ) ;
#13139=DIRECTION ( 'NONE',  ( -0.000000000000000000, -1.000000000000000000, -0.000000000000000000 ) ) ;
#13141=FACE_OUTER_BOUND ( 'NONE', #11844, .T. ) ;
#13176=ORIENTED_EDGE ( 'NONE', *, *, #7433, .F. ) ;
#13194=DIRECTION ( 'NONE',  ( -0.000000000000000000, 1.000000000000000000, -0.000000000000000000 ) ) ;
#13203=DIRECTION ( 'NONE',  ( 0.000000000000000000, -0.000000000000000000, 1.000000000000000000 ) ) ;
#13207=FACE_OUTER_BOUND ( 'NONE', #14143, .T. ) ;
#13211=EDGE_CURVE ( 'NONE', #1645, #4842, #448, .T. ) ;
#13215=LINE ( 'NONE', #4219, #13750 ) ;
#13240=CARTESIAN_POINT ( 'NONE',  ( 60.00000000000000000, -6.123233995736768255E-16, 25.00000000000000000 ) ) ;
#13242=CARTESIAN_POINT ( 'NONE',  ( 22.00000000000000000, 80.00000000000000000, -25.00000000000000000 ) ) ;
#13255=CARTESIAN_POINT ( 'NONE',  ( 19.99999999999999645, 57.00000000000000000, 25.00000000000000000 ) ) ;
#13256=ORIENTED_EDGE ( 'NONE', *, *, #8946, .T. ) ;
#13277=EDGE_CURVE ( 'NONE', #4680, #13498, #5981, .T. ) ;
#13284=ORIENTED_EDGE ( 'NONE', *, *, #3619, .F. ) ;
#13306=ORIENTED_EDGE ( 'NONE', *, *, #1983, .T. ) ;
#13307=ORIENTED_EDGE ( 'NONE', *, *, #161, .F. ) ;
#13308=DIRECTION ( 'NONE',  ( 1.000000000000000000, 1.224646799147353454E-16, -0.000000000000000000 ) ) ;
#13321=VECTOR ( 'NONE', #13767, 1000.000000000000000 ) ;
#13327=ORIENTED_EDGE ( 'NONE', *, *, #6509, .T. ) ;
#13328=ORIENTED_EDGE ( 'NONE', *, *, #5413, .F. ) ;
#13335=DIRECTION ( 'NONE',  ( 0.000000000000000000, 0.000000000000000000, -1.000000000000000000 ) ) ;
#13380=ORIENTED_EDGE ( 'NONE', *, *, #14047, .T. ) ;
#13384=VECTOR ( 'NONE', #6725, 1000.000000000000000 ) ;
#13410=ORIENTED_EDGE ( 'NONE', *, *, #6509, .F. ) ;
#13413=PLANE ( 'NONE',  #13103 ) ;
#13416=VERTEX_POINT ( 'NONE', #7233 ) ;
#13438=VERTEX_POINT ( 'NONE', #6059 ) ;
#13455=ORIENTED_EDGE ( 'NONE', *, *, #8544, .T. ) ;
#13456=ORIENTED_EDGE ( 'NONE', *, *, #13522, .F. ) ;
#13458=EDGE_CURVE ( 'NONE', #4904, #5824, #11709, .T. ) ;
#13474=ORIENTED_EDGE ( 'NONE', *, *, #3923, .T. ) ;
#13488=ORIENTED_EDGE ( 'NONE', *, *, #11548, .T. ) ;
#13498=VERTEX_POINT ( 'NONE', #10964 ) ;
#13518=ORIENTED_EDGE ( 'NONE', *, *, #1647, .T. ) ;
#13522=EDGE_CURVE ( 'NONE', #815, #10977, #3224, .T. ) ;
#13537=EDGE_CURVE ( 'NONE', #5687, #10580, #11052, .T. ) ;
#13568=EDGE_LOOP ( 'NONE', ( #9102, #14352, #2731, #5053 ) ) ;
#13572=FILL_AREA_STYLE_COLOUR ( '', #976 ) ;
#13577=CARTESIAN_POINT ( 'NONE',  ( 22.00000000000000355, 40.00000000000000711, -25.00000000000000000 ) ) ;
#13608=CONICAL_SURFACE ( 'NONE', #11017, 2.100000000000000977, 1.029744258676656754 ) ;
#13609=CARTESIAN_POINT ( 'NONE',  ( 56.99999999999997868, -8.673617379884035472E-16, 25.00000000000000000 ) ) ;
#13641=ORIENTED_EDGE ( 'NONE', *, *, #8616, .T. ) ;
#13655=ORIENTED_EDGE ( 'NONE', *, *, #8337, .T. ) ;
#13659=VERTEX_POINT ( 'NONE', #2983 ) ;
#13700=CARTESIAN_POINT ( 'NONE',  ( 40.00000000000000711, 80.00000000000000000, -25.00000000000000000 ) ) ;
#13716=DIRECTION ( 'NONE',  ( -1.000000000000000000, 0.000000000000000000, 0.000000000000000000 ) ) ;
#13725=ORIENTED_EDGE ( 'NONE', *, *, #2770, .F. ) ;
#13731=VERTEX_POINT ( 'NONE', #5299 ) ;
#13746=PLANE ( 'NONE',  #8619 ) ;
#13750=VECTOR ( 'NONE', #5575, 1000.000000000000114 ) ;
#13767=DIRECTION ( 'NONE',  ( -1.000000000000000000, -0.000000000000000000, -0.000000000000000000 ) ) ;
#13799=ADVANCED_FACE ( 'NONE', ( #2232 ), #3477, .F. ) ;
#13821=DIRECTION ( 'NONE',  ( 0.000000000000000000, 0.000000000000000000, -1.000000000000000000 ) ) ;
#13825=DIRECTION ( 'NONE',  ( 1.000000000000000000, 1.224646799147353454E-16, -0.000000000000000000 ) ) ;
#13832=CARTESIAN_POINT ( 'NONE',  ( 20.00000000000000000, 60.00000000000000711, 25.00000000000000000 ) ) ;
#13836=ORIENTED_EDGE ( 'NONE', *, *, #5830, .T. ) ;
#13843=DIRECTION ( 'NONE',  ( -0.000000000000000000, -1.000000000000000000, -0.000000000000000000 ) ) ;
#13847=FACE_OUTER_BOUND ( 'NONE', #14264, .T. ) ;
#13855=VECTOR ( 'NONE', #1644, 1000.000000000000000 ) ;
#13892=DIRECTION ( 'NONE',  ( 1.000000000000000000, 0.000000000000000000, 0.000000000000000000 ) ) ;
#13913=CARTESIAN_POINT ( 'NONE',  ( 20.00000000000000000, 60.00000000000000711, 25.00000000000000000 ) ) ;
#13931=EDGE_CURVE ( 'NONE', #7235, #3193, #2184, .T. ) ;
#13943=DIRECTION ( 'NONE',  ( -0.000000000000000000, -0.000000000000000000, -1.000000000000000000 ) ) ;
#13953=PLANE ( 'NONE',  #3767 ) ;
#13958=ORIENTED_EDGE ( 'NONE', *, *, #13127, .F. ) ;
#13980=VECTOR ( 'NONE', #11664, 1000.000000000000000 ) ;
#14008=VERTEX_POINT ( 'NONE', #10406 ) ;
#14032=ORIENTED_EDGE ( 'NONE', *, *, #14047, .F. ) ;
#14047=EDGE_CURVE ( 'NONE', #1073, #5455, #12908, .T. ) ;
#14060=DIRECTION ( 'NONE',  ( -0.000000000000000000, -0.000000000000000000, -1.000000000000000000 ) ) ;
#14076=EDGE_CURVE ( 'NONE', #815, #14008, #2961, .T. ) ;
#14097=EDGE_CURVE ( 'NONE', #12770, #13043, #12088, .T. ) ;
#14102=DIRECTION ( 'NONE',  ( 0.000000000000000000, 0.000000000000000000, -1.000000000000000000 ) ) ;
#14107=CARTESIAN_POINT ( 'NONE',  ( 54.35294117647056567, -1.411764705882362358, 23.00000000000000000 ) ) ;
#14110=ADVANCED_FACE ( 'NONE', ( #618 ), #12990, .F. ) ;
#14120=FACE_OUTER_BOUND ( 'NONE', #4448, .T. ) ;
#14124=EDGE_CURVE ( 'NONE', #13438, #14008, #5283, .T. ) ;
#14143=EDGE_LOOP ( 'NONE', ( #6402, #6161, #13488, #9811 ) ) ;
#14155=ADVANCED_FACE ( 'NONE', ( #10907 ), #14292, .T. ) ;
#14165=VERTEX_POINT ( 'NONE', #6229 ) ;
#14168=VERTEX_POINT ( 'NONE', #7680 ) ;
#14176=ORIENTED_EDGE ( 'NONE', *, *, #13522, .T. ) ;
#14179=CARTESIAN_POINT ( 'NONE',  ( 24.99999999999999289, -4.898587196589414604E-15, -25.00000000000000000 ) ) ;
#14197=DIRECTION ( 'NONE',  ( 1.000000000000000000, 1.224646799147353454E-16, -0.000000000000000000 ) ) ;
#14201=CARTESIAN_POINT ( 'NONE',  ( 54.35294117647056567, -1.411764705882362358, 23.00000000000000000 ) ) ;
#14217=EDGE_CURVE ( 'NONE', #3543, #13416, #3323, .T. ) ;
#14219=EDGE_CURVE ( 'NONE', #3170, #10977, #1108, .T. ) ;
#14224=DIRECTION ( 'NONE',  ( 0.000000000000000000, 0.000000000000000000, -1.000000000000000000 ) ) ;
#14259=ORIENTED_EDGE ( 'NONE', *, *, #12907, .F. ) ;
#14264=EDGE_LOOP ( 'NONE', ( #9009, #10556, #2435, #14259 ) ) ;
#14278=CARTESIAN_POINT ( 'NONE',  ( 22.00000000000000711, 20.00000000000000355, 25.00000000000000000 ) ) ;
#14279=EDGE_CURVE ( 'NONE', #10817, #4904, #1041, .T. ) ;
#14292=PLANE ( 'NONE',  #11514 ) ;
#14306=VERTEX_POINT ( 'NONE', #10419 ) ;
#14316=EDGE_CURVE ( 'NONE', #1016, #4305, #3924, .T. ) ;
#14319=CARTESIAN_POINT ( 'NONE',  ( 36.99999999999999289, 80.00000000000000000, 25.00000000000000000 ) ) ;
#14320=ORIENTED_EDGE ( 'NONE', *, *, #8337, .F. ) ;
#14322=DIRECTION ( 'NONE',  ( -1.224646799147353454E-16, 1.000000000000000000, 0.000000000000000000 ) ) ;
#14327=ORIENTED_EDGE ( 'NONE', *, *, #12907, .T. ) ;
#14352=ORIENTED_EDGE ( 'NONE', *, *, #6443, .T. ) ;
#14366=EDGE_CURVE ( 'NONE', #12770, #1645, #560, .T. ) ;
#14374=CARTESIAN_POINT ( 'NONE',  ( 20.00000000000000355, 30.00000000000000711, 25.00000000000000000 ) ) ;
#14380=ORIENTED_EDGE ( 'NONE', *, *, #4547, .F. ) ;
#14428=ORIENTED_EDGE ( 'NONE', *, *, #8544, .F. ) ;
#14429=DIRECTION ( 'NONE',  ( -0.000000000000000000, 0.000000000000000000, 1.000000000000000000 ) ) ;
#14430=CARTESIAN_POINT ( 'NONE',  ( 22.00000000000000355, 40.00000000000000711, -25.00000000000000000 ) ) ;
#14431=CYLINDRICAL_SURFACE ( 'NONE', #511, 2.100000000000000977 ) ;
#14433=ORIENTED_EDGE ( 'NONE', *, *, #4070, .F. ) ;
#14443=EDGE_CURVE ( 'NONE', #721, #7705, #11969, .T. ) ;
#14453=CARTESIAN_POINT ( 'NONE',  ( 54.35294117647056567, -1.411764705882362358, -23.00000000000000000 ) ) ;
#14461=CARTESIAN_POINT ( 'NONE',  ( 20.00000000000000000, 80.00000000000000000, -25.00000000000000000 ) ) ;
#14463=EDGE_LOOP ( 'NONE', ( #6066, #13327, #5213, #2389 ) ) ;
ENDSEC;
END-ISO-10303-21;
